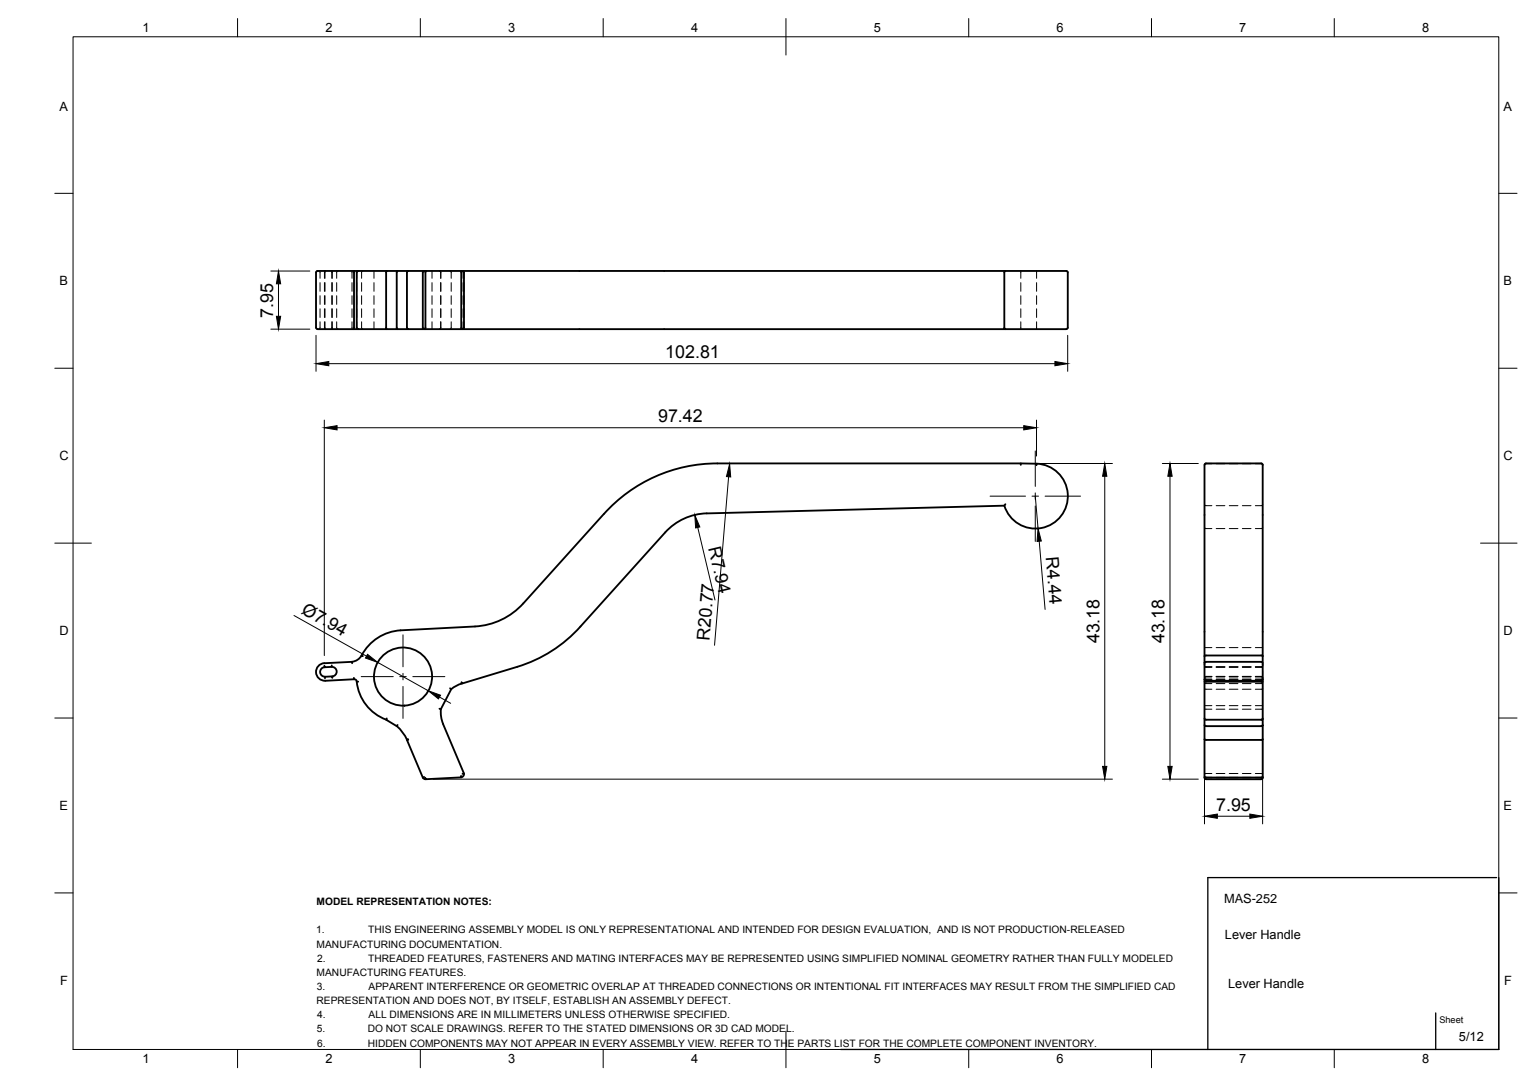
ISO-10303-21;
HEADER;
FILE_DESCRIPTION((''),'2;1');
FILE_NAME('Lever Handle.step','2026-10-06T07:01:46+05:00',(''),(''),'','','');
FILE_SCHEMA (('AUTOMOTIVE_DESIGN { 1 0 10303 214 3 1 1 }'));
ENDSEC;
DATA;
#10=MECHANICAL_DESIGN_GEOMETRIC_PRESENTATION_REPRESENTATION('',(#140),#11396);
#106=(
BOUNDED_SURFACE()
B_SPLINE_SURFACE(2,2,((#9482,#9483,#9484),(#9485,#9486,#9487),(#9488,#9489,
#9490)),.UNSPECIFIED.,.F.,.F.,.F.)
B_SPLINE_SURFACE_WITH_KNOTS((3,3),(3,3),(0.,1.5707963267949),(-2.95294089690097,
-1.43909013515432),.UNSPECIFIED.)
GEOMETRIC_REPRESENTATION_ITEM()
RATIONAL_B_SPLINE_SURFACE(((1.,0.726950752418356,1.),(0.707106781186548,
0.514031806623683,0.707106781186548),(1.,0.726950752418356,1.)))
REPRESENTATION_ITEM('')
SURFACE()
) ;
#107=(
BOUNDED_SURFACE()
B_SPLINE_SURFACE(2,2,((#10602,#10603,#10604),(#10605,#10606,#10607),(#10608,
#10609,#10610)),.UNSPECIFIED.,.F.,.F.,.F.)
B_SPLINE_SURFACE_WITH_KNOTS((3,3),(3,3),(-1.5707963267949,0.),(-2.95294089690006,
-1.43909013515442),.UNSPECIFIED.)
GEOMETRIC_REPRESENTATION_ITEM()
RATIONAL_B_SPLINE_SURFACE(((1.,0.726950752418703,1.),(0.707106781186561,
0.514031806623938,0.707106781186561),(1.,0.726950752418703,1.)))
REPRESENTATION_ITEM('')
SURFACE()
) ;
#110=SHAPE_REPRESENTATION_RELATIONSHIP('SRR','None',#11457,#125) ;
#125=ADVANCED_BREP_SHAPE_REPRESENTATION('',(#155),#11383) ;
#140=STYLED_ITEM('',(#11541),#155) ;
#155=MANIFOLD_SOLID_BREP('Lever Handle',#5571) ;
#202=TOROIDAL_SURFACE('',#6043,5.6095419988581,0.2) ;
#203=TOROIDAL_SURFACE('',#6047,18.7717409779691,0.2) ;
#204=TOROIDAL_SURFACE('',#6051,6.02789861439302,0.2) ;
#205=TOROIDAL_SURFACE('',#6055,0.524935224963979,0.2) ;
#206=TOROIDAL_SURFACE('',#6061,1.8962519345458,0.2) ;
#207=TOROIDAL_SURFACE('',#6064,20.567808830506,0.2) ;
#208=TOROIDAL_SURFACE('',#6067,6.24675996480776,0.2) ;
#209=TOROIDAL_SURFACE('',#6070,9.77267576253889,0.2) ;
#210=TOROIDAL_SURFACE('',#6077,1.00004201680672,0.2) ;
#211=TOROIDAL_SURFACE('',#6080,4.23606098801213,0.2) ;
#212=TOROIDAL_SURFACE('',#6084,8.13937148944777,0.2) ;
#213=TOROIDAL_SURFACE('',#6089,3.96067266925812,0.2) ;
#214=TOROIDAL_SURFACE('',#6093,4.37909654020415,0.2) ;
#215=TOROIDAL_SURFACE('',#6097,0.274381812079108,0.2) ;
#216=TOROIDAL_SURFACE('',#6128,0.274381812079108,0.2) ;
#217=TOROIDAL_SURFACE('',#6131,4.37909654020415,0.2) ;
#218=TOROIDAL_SURFACE('',#6135,3.96067266925812,0.2) ;
#219=TOROIDAL_SURFACE('',#6139,8.13937148944777,0.2) ;
#220=TOROIDAL_SURFACE('',#6144,1.00004201680672,0.2) ;
#221=TOROIDAL_SURFACE('',#6146,4.23606098801213,0.2) ;
#222=TOROIDAL_SURFACE('',#6151,9.77267576253889,0.2) ;
#223=TOROIDAL_SURFACE('',#6156,20.567808830506,0.2) ;
#224=TOROIDAL_SURFACE('',#6159,6.24675996480776,0.2) ;
#225=TOROIDAL_SURFACE('',#6162,1.8962519345458,0.2) ;
#226=TOROIDAL_SURFACE('',#6166,0.524935224963979,0.2) ;
#227=TOROIDAL_SURFACE('',#6169,18.7717409779691,0.2) ;
#228=TOROIDAL_SURFACE('',#6172,6.02789861439302,0.2) ;
#229=TOROIDAL_SURFACE('',#6175,5.6095419988581,0.2) ;
#230=TOROIDAL_SURFACE('',#6199,0.85017716535433,0.2) ;
#231=TOROIDAL_SURFACE('',#6202,0.85017716535433,0.2) ;
#232=TOROIDAL_SURFACE('',#6207,0.85017716535433,0.2) ;
#233=TOROIDAL_SURFACE('',#6209,0.85017716535433,0.2) ;
#271=B_SPLINE_CURVE_WITH_KNOTS('',3,(#9456,#9457,#9458,#9459,#9460,#9461,
#9462,#9463,#9464,#9465,#9466,#9467),.UNSPECIFIED.,.F.,.F.,(4,2,2,2,2,4),
(-0.000425934342717597,0.,0.00767782768113804,0.0154936481323793,0.0233033297268441,
0.0311102612476663),.UNSPECIFIED.) ;
#272=B_SPLINE_CURVE_WITH_KNOTS('',3,(#9470,#9471,#9472,#9473,#9474,#9475,
#9476,#9477,#9478,#9479,#9480,#9481),.UNSPECIFIED.,.F.,.F.,(4,2,2,2,2,4),
(-0.000392646763472729,0.,0.00776851635729194,0.0155945832419373,0.0233973193253328,
0.0311896776950334),.UNSPECIFIED.) ;
#273=B_SPLINE_CURVE_WITH_KNOTS('',3,(#9494,#9495,#9496,#9497,#9498,#9499,
#9500,#9501,#9502,#9503,#9504,#9505),.UNSPECIFIED.,.F.,.F.,(4,2,2,2,2,4),
(-0.0626678583597519,-0.0622419978775531,-0.0545506208202995,-0.046733489174686,
-0.0389252522766465,-0.0311209989394379),.UNSPECIFIED.) ;
#274=B_SPLINE_CURVE_WITH_KNOTS('',3,(#9511,#9512,#9513,#9514,#9515,#9516,
#9517,#9518,#9519,#9520,#9521,#9522),.UNSPECIFIED.,.F.,.F.,(4,2,2,2,2,4),
(-0.00029630356009181,0.,0.00778002873103429,0.0155932483092341,0.0234059593652307,
0.0312184094334333),.UNSPECIFIED.) ;
#275=B_SPLINE_CURVE_WITH_KNOTS('',3,(#9528,#9529,#9530,#9531,#9532,#9533,
#9534,#9535,#9536,#9537,#9538,#9539),.UNSPECIFIED.,.F.,.F.,(4,2,2,2,2,4),
(-0.0629385074257631,-0.0627334798904802,-0.0547568943966375,-0.046925593190769,
-0.0391229130222982,-0.0313664342990436),.UNSPECIFIED.) ;
#276=B_SPLINE_CURVE_WITH_KNOTS('',3,(#9545,#9546,#9547,#9548,#9549,#9550,
#9551,#9552,#9553,#9554,#9555,#9556),.UNSPECIFIED.,.F.,.F.,(4,2,2,2,2,4),
(-0.000203756697037429,0.,0.00796770405795475,0.0158037932485574,0.0236037819491495,
0.031385705039184),.UNSPECIFIED.) ;
#277=B_SPLINE_CURVE_WITH_KNOTS('',3,(#9561,#9562,#9563,#9564,#9565,#9566,
#9567,#9568,#9569,#9570,#9571,#9572,#9573,#9574,#9575,#9576,#9577,#9578,
#9579,#9580,#9581,#9582,#9583,#9584,#9585),.UNSPECIFIED.,.F.,.F.,(4,3,3,
3,3,3,3,3,4),(0.,0.199052542232163,0.398059502796862,0.597027074925485,
0.795961438809451,0.995008849549264,1.19397259651743,1.39300992499601,1.57079632692443),
 .UNSPECIFIED.) ;
#278=B_SPLINE_CURVE_WITH_KNOTS('',3,(#9589,#9590,#9591,#9592,#9593,#9594,
#9595,#9596,#9597,#9598,#9599,#9600),.UNSPECIFIED.,.F.,.F.,(4,2,2,2,2,4),
(-0.000302162807502731,0.,0.00777281639954654,0.0155857029470102,0.0233985882068449,
0.0312114728139599),.UNSPECIFIED.) ;
#279=B_SPLINE_CURVE_WITH_KNOTS('',3,(#9607,#9608,#9609,#9610,#9611,#9612,
#9613,#9614,#9615,#9616,#9617,#9618),.UNSPECIFIED.,.F.,.F.,(4,2,2,2,2,4),
(-0.0315148928540183,-0.0312005996265522,-0.0234381588919511,-0.0156248125751573,
-0.00781221363393156,0.),.UNSPECIFIED.) ;
#280=B_SPLINE_CURVE_WITH_KNOTS('',3,(#9623,#9624,#9625,#9626,#9627,#9628,
#9629,#9630,#9631,#9632,#9633,#9634),.UNSPECIFIED.,.F.,.F.,(4,2,2,2,2,4),
(-0.000209158996821947,0.,0.00790322324693375,0.0157271724669949,0.0235347393467978,
0.0313323503074072),.UNSPECIFIED.) ;
#281=B_SPLINE_CURVE_WITH_KNOTS('',3,(#9640,#9641,#9642,#9643,#9644,#9645,
#9646,#9647,#9648,#9649,#9650,#9651,#9652,#9653,#9654,#9655,#9656,#9657,
#9658,#9659,#9660,#9661,#9662,#9663,#9664),.UNSPECIFIED.,.F.,.F.,(4,3,3,
3,3,3,3,3,4),(0.,0.199052706978784,0.398059832253966,0.597027569062776,
0.7959620976022,0.99500967309516,1.19397358474941,1.39301107797699,1.57079762660799),
 .UNSPECIFIED.) ;
#282=B_SPLINE_CURVE_WITH_KNOTS('',3,(#9670,#9671,#9672,#9673,#9674,#9675,
#9676,#9677,#9678,#9679,#9680,#9681),.UNSPECIFIED.,.F.,.F.,(4,2,2,2,2,4),
(-0.000508786942166875,0.,0.00757813380105505,0.0153951238953111,0.0232058288277231,
0.0310129102887088),.UNSPECIFIED.) ;
#283=B_SPLINE_CURVE_WITH_KNOTS('',3,(#9686,#9687,#9688,#9689,#9690,#9691,
#9692,#9693,#9694,#9695,#9696,#9697,#9698,#9699,#9700,#9701,#9702,#9703,
#9704,#9705,#9706,#9707,#9708,#9709,#9710),.UNSPECIFIED.,.F.,.F.,(4,3,3,
3,3,3,3,3,4),(0.,0.199053248397837,0.398060914968089,0.597029192964828,
0.79596426260186,0.995012379499913,1.1939768323317,1.39301486693695,1.57080189914441),
 .UNSPECIFIED.) ;
#284=B_SPLINE_CURVE_WITH_KNOTS('',3,(#9714,#9715,#9716,#9717,#9718,#9719,
#9720,#9721,#9722,#9723,#9724,#9725,#9726,#9727,#9728,#9729),
 .UNSPECIFIED.,.F.,.F.,(4,2,2,2,2,2,2,4),(-0.00032358937009677,0.,0.00354444219611517,
0.00767686671153501,0.0154916858096829,0.0233035611079842,0.0311138771958668,
0.0311774645866534),.UNSPECIFIED.) ;
#285=B_SPLINE_CURVE_WITH_KNOTS('',3,(#9736,#9737,#9738,#9739,#9740,#9741,
#9742,#9743,#9744,#9745,#9746,#9747,#9748,#9749,#9750,#9751,#9752,#9753,
#9754,#9755,#9756,#9757,#9758,#9759,#9760),.UNSPECIFIED.,.F.,.F.,(4,3,3,
3,3,3,3,3,4),(0.,0.199052583563084,0.398059585450825,0.597027198896615,
0.795961604093608,0.99500905617405,1.19397284446766,1.39301021428897,1.57079665269337),
 .UNSPECIFIED.) ;
#286=B_SPLINE_CURVE_WITH_KNOTS('',3,(#9768,#9769,#9770,#9771,#9772,#9773,
#9774,#9775,#9776,#9777,#9778,#9779),.UNSPECIFIED.,.F.,.F.,(4,2,2,2,2,4),
(-0.0315123462948468,-0.031000483210486,-0.0234384406752481,-0.0156253470993035,
-0.00781258687358792,0.),.UNSPECIFIED.) ;
#287=B_SPLINE_CURVE_WITH_KNOTS('',3,(#9785,#9786,#9787,#9788,#9789,#9790,
#9791,#9792,#9793,#9794,#9795,#9796,#9797,#9798,#9799,#9800,#9801,#9802,
#9803,#9804,#9805,#9806,#9807,#9808,#9809),.UNSPECIFIED.,.F.,.F.,(4,3,3,
3,3,3,3,3,4),(0.,0.199052542245368,0.398059502823902,0.59702707496727,0.795961438867092,
0.9950088496244,1.19397259661093,1.39300992510867,1.57079632687287),
 .UNSPECIFIED.) ;
#288=B_SPLINE_CURVE_WITH_KNOTS('',3,(#9815,#9816,#9817,#9818,#9819,#9820,
#9821,#9822,#9823,#9824,#9825,#9826),.UNSPECIFIED.,.F.,.F.,(4,2,2,2,2,4),
(-0.000472807702419667,0.,0.00760072048225168,0.0154136353110866,0.0232265107396055,
0.0310393663455244),.UNSPECIFIED.) ;
#289=B_SPLINE_CURVE_WITH_KNOTS('',3,(#9831,#9832,#9833,#9834,#9835,#9836,
#9837,#9838,#9839,#9840,#9841,#9842,#9843,#9844,#9845,#9846,#9847,#9848,
#9849,#9850,#9851,#9852,#9853,#9854,#9855),.UNSPECIFIED.,.F.,.F.,(4,3,3,
3,3,3,3,3,4),(0.,0.199052542243981,0.398059502821061,0.597027074962877,
0.795961438861017,0.995008849616485,1.19397259660109,1.39300992509683,1.57079632687829),
 .UNSPECIFIED.) ;
#290=B_SPLINE_CURVE_WITH_KNOTS('',3,(#9872,#9873,#9874,#9875,#9876,#9877,
#9878,#9879,#9880,#9881,#9882,#9883),.UNSPECIFIED.,.F.,.F.,(4,2,2,2,2,4),
(-0.0315141126684919,-0.031176944954667,-0.0234383818709659,-0.0156252430234338,
-0.00781251789292829,0.),.UNSPECIFIED.) ;
#291=B_SPLINE_CURVE_WITH_KNOTS('',3,(#9887,#9888,#9889,#9890,#9891,#9892,
#9893,#9894,#9895,#9896,#9897,#9898,#9899,#9900,#9901,#9902,#9903,#9904,
#9905,#9906,#9907,#9908,#9909,#9910,#9911),.UNSPECIFIED.,.F.,.F.,(4,3,3,
3,3,3,3,3,4),(0.,0.199052485193076,0.398059386004224,0.597026894426605,
0.795961189880508,0.995008525064052,1.19397219273933,1.39300943847609,1.57079654966886),
 .UNSPECIFIED.) ;
#292=B_SPLINE_CURVE_WITH_KNOTS('',3,(#9919,#9920,#9921,#9922,#9923,#9924,
#9925,#9926,#9927,#9928,#9929,#9930,#9931,#9932),.UNSPECIFIED.,.F.,.F.,
(4,2,2,2,2,2,4),(-0.071485180683264,-0.0712307719726932,-0.064253173333706,
-0.0574900962687512,-0.0489313629526751,-0.0419539746827257,-0.0356153859867279),
 .UNSPECIFIED.) ;
#293=B_SPLINE_CURVE_WITH_KNOTS('',3,(#9950,#9951,#9952,#9953,#9954,#9955,
#9956,#9957,#9958,#9959,#9960,#9961,#9962,#9963),.UNSPECIFIED.,.F.,.F.,
(4,2,2,2,2,2,4),(-0.063419024433945,-0.0632138433555934,-0.0550363404792558,
-0.0471273977752151,-0.0393668335371398,-0.0316820163148599,-0.0316075730538707),
 .UNSPECIFIED.) ;
#294=B_SPLINE_CURVE_WITH_KNOTS('',3,(#9969,#9970,#9971,#9972,#9973,#9974,
#9975,#9976,#9977,#9978,#9979,#9980,#9981,#9982),.UNSPECIFIED.,.F.,.F.,
(4,2,2,2,2,2,4),(-0.000204835146312565,0.,0.00817143806143788,0.0160775285373022,
0.0238394400759123,0.0315278536559536,0.0315985683409222),.UNSPECIFIED.) ;
#295=B_SPLINE_CURVE_WITH_KNOTS('',3,(#9987,#9988,#9989,#9990,#9991,#9992,
#9993,#9994,#9995,#9996,#9997,#9998,#9999,#10000),.UNSPECIFIED.,.F.,.F.,
(4,2,2,2,2,2,4),(-0.0315119651507534,-0.0310369720406695,-0.0234522322979694,
-0.0156393394528541,-0.00782644846731675,-1.35584415946594E-5,0.),
 .UNSPECIFIED.) ;
#296=B_SPLINE_CURVE_WITH_KNOTS('',3,(#10007,#10008,#10009,#10010,#10011,
#10012,#10013,#10014,#10015,#10016,#10017,#10018),.UNSPECIFIED.,.F.,.F.,
(4,2,2,2,2,4),(-0.031721691652862,-0.0314189347322439,-0.0233633267396854,
-0.0155133765946492,-0.00773979585571865,0.),.UNSPECIFIED.) ;
#297=B_SPLINE_CURVE_WITH_KNOTS('',3,(#10099,#10100,#10101,#10102,#10103,
#10104,#10105,#10106,#10107,#10108,#10109,#10110),.UNSPECIFIED.,.F.,.F.,
(4,2,2,2,2,4),(-0.000302979244329871,0.,0.00806152347440571,0.0159172380801614,
0.0236965271994009,0.0314420066261495),.UNSPECIFIED.) ;
#298=B_SPLINE_CURVE_WITH_KNOTS('',3,(#10111,#10112,#10113,#10114,#10115,
#10116,#10117,#10118,#10119,#10120,#10121,#10122),.UNSPECIFIED.,.F.,.F.,
(4,2,2,2,2,4),(-0.0315754136058091,-0.0311828527614278,-0.0234160363129251,
-0.0155916819303375,-0.00779065324374899,0.),.UNSPECIFIED.) ;
#299=B_SPLINE_CURVE_WITH_KNOTS('',3,(#10127,#10128,#10129,#10130,#10131,
#10132,#10133,#10134,#10135,#10136,#10137,#10138,#10139,#10140),
 .UNSPECIFIED.,.F.,.F.,(4,2,2,2,2,2,4),(-0.000474992982336123,0.,0.00758473725973339,
0.0153976269864644,0.0232105148526209,0.0310234017590763,0.0310369601957522),
 .UNSPECIFIED.) ;
#300=B_SPLINE_CURVE_WITH_KNOTS('',3,(#10146,#10147,#10148,#10149,#10150,
#10151,#10152,#10153,#10154,#10155,#10156,#10157),.UNSPECIFIED.,.F.,.F.,
(4,2,2,2,2,4),(-0.0634032075025796,-0.0631983745559419,-0.0551219653781809,
-0.0471164301307063,-0.039256298781182,-0.0315985683616453),
 .UNSPECIFIED.) ;
#301=B_SPLINE_CURVE_WITH_KNOTS('',3,(#10163,#10164,#10165,#10166,#10167,
#10168,#10169,#10170,#10171,#10172,#10173,#10174),.UNSPECIFIED.,.F.,.F.,
(4,2,2,2,2,4),(-0.000205178731636372,0.,0.00808313825878162,0.0160941684934645,
0.0239559117961846,0.0316075730471855),.UNSPECIFIED.) ;
#302=B_SPLINE_CURVE_WITH_KNOTS('',3,(#10180,#10181,#10182,#10183,#10184,
#10185,#10186,#10187,#10188,#10189,#10190,#10191),.UNSPECIFIED.,.F.,.F.,
(4,2,2,2,2,4),(-0.000314294385248188,0.,0.00776246933425461,0.0155758444397962,
0.0233884721670194,0.0312007145855276),.UNSPECIFIED.) ;
#303=B_SPLINE_CURVE_WITH_KNOTS('',3,(#10195,#10196,#10197,#10198,#10199,
#10200,#10201,#10202,#10203,#10204,#10205,#10206,#10207,#10208,#10209,#10210,
#10211,#10212,#10213,#10214,#10215,#10216,#10217,#10218,#10219),
 .UNSPECIFIED.,.F.,.F.,(4,3,3,3,3,3,3,3,4),(0.,0.199053248397837,0.398060914968088,
0.597029192964836,0.795964262601867,0.995012379499923,1.19397683233171,
1.39301486693695,1.57080189914441),.UNSPECIFIED.) ;
#304=B_SPLINE_CURVE_WITH_KNOTS('',3,(#10222,#10223,#10224,#10225,#10226,
#10227,#10228,#10229,#10230,#10231,#10232,#10233),.UNSPECIFIED.,.F.,.F.,
(4,2,2,2,2,4),(-0.0315210097541554,-0.0310122339084761,-0.0234342653837737,
-0.0156174457752067,-0.00780691119140275,0.),.UNSPECIFIED.) ;
#305=B_SPLINE_CURVE_WITH_KNOTS('',3,(#10237,#10238,#10239,#10240,#10241,
#10242,#10243,#10244,#10245,#10246,#10247,#10248,#10249,#10250,#10251,#10252,
#10253,#10254,#10255,#10256,#10257,#10258,#10259,#10260,#10261),
 .UNSPECIFIED.,.F.,.F.,(4,3,3,3,3,3,3,3,4),(0.,0.199052542064369,0.398059502453293,
0.597027074394497,0.795961438077169,0.995008848594717,1.19397259532962,
1.39300992356481,1.57079632757971),.UNSPECIFIED.) ;
#306=B_SPLINE_CURVE_WITH_KNOTS('',3,(#10272,#10273,#10274,#10275,#10276,
#10277,#10278,#10279,#10280,#10281,#10282,#10283,#10284,#10285),
 .UNSPECIFIED.,.F.,.F.,(4,2,2,2,2,2,4),(-0.000254408710349561,0.,0.00697759863796767,
0.0137406757011616,0.0222994090150433,0.0292767972832062,0.035615385977577),
 .UNSPECIFIED.) ;
#307=B_SPLINE_CURVE_WITH_KNOTS('',3,(#10288,#10289,#10290,#10291,#10292,
#10293,#10294,#10295,#10296,#10297,#10298,#10299,#10300,#10301,#10302,#10303,
#10304,#10305,#10306,#10307,#10308,#10309,#10310,#10311,#10312),
 .UNSPECIFIED.,.F.,.F.,(4,3,3,3,3,3,3,3,4),(0.,0.199052485193076,0.398059386004222,
0.597026894426605,0.795961189880508,0.995008525064048,1.19397219273933,
1.39300943847609,1.57079654966886),.UNSPECIFIED.) ;
#308=B_SPLINE_CURVE_WITH_KNOTS('',3,(#10318,#10319,#10320,#10321,#10322,
#10323,#10324,#10325,#10326,#10327,#10328,#10329),.UNSPECIFIED.,.F.,.F.,
(4,2,2,2,2,4),(-0.000337168458022535,0.,0.00773858016387553,0.0155517362556591,
0.0233644786295,0.031177013765312),.UNSPECIFIED.) ;
#309=B_SPLINE_CURVE_WITH_KNOTS('',3,(#10339,#10340,#10341,#10342,#10343,
#10344,#10345,#10346,#10347,#10348,#10349,#10350,#10351,#10352,#10353,#10354,
#10355,#10356,#10357,#10358,#10359,#10360,#10361,#10362,#10363),
 .UNSPECIFIED.,.F.,.F.,(4,3,3,3,3,3,3,3,4),(0.,0.199052542234199,0.398059502803477,
0.597027074940396,0.795961438837137,0.995008849596832,1.1939725965883,1.39300992509389,
1.57079632687829),.UNSPECIFIED.) ;
#310=B_SPLINE_CURVE_WITH_KNOTS('',3,(#10370,#10371,#10372,#10373,#10374,
#10375,#10376,#10377,#10378,#10379,#10380,#10381,#10382,#10383,#10384,#10385,
#10386,#10387,#10388,#10389,#10390,#10391,#10392,#10393,#10394),
 .UNSPECIFIED.,.F.,.F.,(4,3,3,3,3,3,3,3,4),(0.,0.199052646770473,0.398059711851129,
0.597027388477328,0.795961856844187,0.99500937213039,1.19397322360319,1.39301065662705,
1.5707971514832),.UNSPECIFIED.) ;
#311=B_SPLINE_CURVE_WITH_KNOTS('',3,(#10400,#10401,#10402,#10403,#10404,
#10405,#10406,#10407,#10408,#10409,#10410,#10411),.UNSPECIFIED.,.F.,.F.,
(4,2,2,2,2,4),(-0.0315121677712463,-0.0310393601655826,-0.0234386412048373,
-0.0156257279288386,-0.00781285405311264,0.),.UNSPECIFIED.) ;
#312=B_SPLINE_CURVE_WITH_KNOTS('',3,(#10415,#10416,#10417,#10418,#10419,
#10420,#10421,#10422,#10423,#10424,#10425,#10426,#10427,#10428,#10429,#10430,
#10431,#10432,#10433,#10434,#10435,#10436,#10437,#10438,#10439),
 .UNSPECIFIED.,.F.,.F.,(4,3,3,3,3,3,3,3,4),(0.,0.199052542257445,0.39805950284863,
0.597027075005487,0.795961438919784,0.995008849693087,1.1939725966964,1.39300992521166,
1.57079632682576),.UNSPECIFIED.) ;
#313=B_SPLINE_CURVE_WITH_KNOTS('',3,(#10445,#10446,#10447,#10448,#10449,
#10450,#10451,#10452,#10453,#10454,#10455,#10456),.UNSPECIFIED.,.F.,.F.,
(4,2,2,2,2,4),(-0.0315141739942469,-0.031204434348752,-0.0234384419466034,
-0.0156253478250137,-0.00781258702147206,0.),.UNSPECIFIED.) ;
#314=B_SPLINE_CURVE_WITH_KNOTS('',3,(#10463,#10464,#10465,#10466,#10467,
#10468,#10469,#10470,#10471,#10472,#10473,#10474),.UNSPECIFIED.,.F.,.F.,
(4,2,2,2,2,4),(-0.0626970871191847,-0.0623734982158925,-0.054555633082751,
-0.0467389670549674,-0.0389250691737583,-0.0311774645911791),
 .UNSPECIFIED.) ;
#315=B_SPLINE_CURVE_WITH_KNOTS('',3,(#10480,#10481,#10482,#10483,#10484,
#10485,#10486,#10487,#10488,#10489,#10490,#10491,#10492,#10493,#10494,#10495,
#10496,#10497,#10498,#10499,#10500,#10501,#10502,#10503,#10504),
 .UNSPECIFIED.,.F.,.F.,(4,3,3,3,3,3,3,3,4),(0.,0.199052686881998,0.398059792064997,
0.597027508785601,0.795962017240172,0.995009572636864,1.1939734642033,1.39301093733562,
1.57079746801826),.UNSPECIFIED.) ;
#316=B_SPLINE_CURVE_WITH_KNOTS('',3,(#10510,#10511,#10512,#10513,#10514,
#10515,#10516,#10517,#10518,#10519,#10520,#10521),.UNSPECIFIED.,.F.,.F.,
(4,2,2,2,2,4),(-0.000404724526048245,0.,0.00770679420177707,0.015530569118343,
0.0233375581471532,0.0311349644051186),.UNSPECIFIED.) ;
#317=B_SPLINE_CURVE_WITH_KNOTS('',3,(#10526,#10527,#10528,#10529,#10530,
#10531,#10532,#10533,#10534,#10535,#10536,#10537),.UNSPECIFIED.,.F.,.F.,
(4,2,2,2,2,4),(-0.0315136505422076,-0.0312114875916089,-0.0234386675146469,
-0.0156257772666477,-0.00781288830710044,0.),.UNSPECIFIED.) ;
#318=B_SPLINE_CURVE_WITH_KNOTS('',3,(#10545,#10546,#10547,#10548,#10549,
#10550,#10551,#10552,#10553,#10554,#10555,#10556),.UNSPECIFIED.,.F.,.F.,
(4,2,2,2,2,4),(-0.0629751667751677,-0.0627714100781202,-0.0548037060202023,
-0.0469676168296412,-0.0391676281290893,-0.0313857050390938),
 .UNSPECIFIED.) ;
#319=B_SPLINE_CURVE_WITH_KNOTS('',3,(#10560,#10561,#10562,#10563,#10564,
#10565,#10566,#10567,#10568,#10569,#10570,#10571),.UNSPECIFIED.,.F.,.F.,
(4,2,2,2,2,4),(-0.00020502755219765,0.,0.00797658615153273,0.015807888001696,
0.0236105688121075,0.031367048172),.UNSPECIFIED.) ;
#320=B_SPLINE_CURVE_WITH_KNOTS('',3,(#10575,#10576,#10577,#10578,#10579,
#10580,#10581,#10582,#10583,#10584,#10585,#10586),.UNSPECIFIED.,.F.,.F.,
(4,2,2,2,2,4),(-0.0315146329369706,-0.0312183301295434,-0.0234383211620277,
-0.0156251214317014,-0.00781243022228811,0.),.UNSPECIFIED.) ;
#321=B_SPLINE_CURVE_WITH_KNOTS('',3,(#10590,#10591,#10592,#10593,#10594,
#10595,#10596,#10597,#10598,#10599,#10600,#10601),.UNSPECIFIED.,.F.,.F.,
(4,2,2,2,2,4),(-0.00042586048217451,0.,0.00769137706195492,0.0155085087115375,
0.0233167456135432,0.0311209989547217),.UNSPECIFIED.) ;
#322=B_SPLINE_CURVE_WITH_KNOTS('',3,(#10613,#10614,#10615,#10616,#10617,
#10618,#10619,#10620,#10621,#10622,#10623,#10624),.UNSPECIFIED.,.F.,.F.,
(4,2,2,2,2,4),(-0.0626464568378844,-0.0622205224951688,-0.0545426948140428,
-0.0467268743628218,-0.038917192768381,-0.0311102612475827),
 .UNSPECIFIED.) ;
#323=B_SPLINE_CURVE_WITH_KNOTS('',3,(#10667,#10668,#10669,#10670,#10671,
#10672,#10673,#10674,#10675,#10676,#10677,#10678),.UNSPECIFIED.,.F.,.F.,
(4,2,2,2,2,4),(-0.000583318373026515,0.,0.00749040753634202,0.0153036497211779,
0.0231163526509165,0.0309287602356685),.UNSPECIFIED.) ;
#324=B_SPLINE_CURVE_WITH_KNOTS('',3,(#10681,#10682,#10683,#10684,#10685,
#10686,#10687,#10688,#10689,#10690,#10691,#10692),.UNSPECIFIED.,.F.,.F.,
(4,2,2,2,2,4),(-0.0315120082952079,-0.0309286912237509,-0.0234383004008955,
-0.0156250756498918,-0.00781239015278319,0.),.UNSPECIFIED.) ;
#325=B_SPLINE_CURVE_WITH_KNOTS('',3,(#10695,#10696,#10697,#10698,#10699,
#10700,#10701,#10702,#10703,#10704,#10705,#10706),.UNSPECIFIED.,.F.,.F.,
(4,2,2,2,2,4),(-0.0315120082952136,-0.0309286912237554,-0.0234383004008859,
-0.0156250756498869,-0.0078123901527818,0.),.UNSPECIFIED.) ;
#326=B_SPLINE_CURVE_WITH_KNOTS('',3,(#10710,#10711,#10712,#10713,#10714,
#10715,#10716,#10717,#10718,#10719,#10720,#10721),.UNSPECIFIED.,.F.,.F.,
(4,2,2,2,2,4),(-0.000583318373025772,0.,0.0074904075363243,0.0153036497211384,
0.0231163526508542,0.0309287602355855),.UNSPECIFIED.) ;
#327=B_SPLINE_CURVE_WITH_KNOTS('',3,(#10738,#10739,#10740,#10741,#10742,
#10743,#10744,#10745,#10746,#10747,#10748,#10749),.UNSPECIFIED.,.F.,.F.,
(4,2,2,2,2,4),(-0.030928760235604,-0.0231163526508699,-0.0153036497211549,
-0.00749040753633595,0.,0.000583318373037331),.UNSPECIFIED.) ;
#328=B_SPLINE_CURVE_WITH_KNOTS('',3,(#10750,#10751,#10752,#10753,#10754,
#10755,#10756,#10757,#10758,#10759,#10760,#10761),.UNSPECIFIED.,.F.,.F.,
(4,2,2,2,2,4),(-0.0315120082952245,-0.0309286912237537,-0.0234383004008807,
-0.0156250756498813,-0.00781239015277872,0.),.UNSPECIFIED.) ;
#329=B_SPLINE_CURVE_WITH_KNOTS('',3,(#10763,#10764,#10765,#10766,#10767,
#10768,#10769,#10770,#10771,#10772,#10773,#10774),.UNSPECIFIED.,.F.,.F.,
(4,2,2,2,2,4),(-0.0315120082952178,-0.0309286912237491,-0.0234383004008884,
-0.0156250756498874,-0.00781239015278138,0.),.UNSPECIFIED.) ;
#330=B_SPLINE_CURVE_WITH_KNOTS('',3,(#10775,#10776,#10777,#10778,#10779,
#10780,#10781,#10782,#10783,#10784,#10785,#10786),.UNSPECIFIED.,.F.,.F.,
(4,2,2,2,2,4),(-0.00058331837303795,0.,0.00749040753635054,0.0153036497211894,
0.0231163526509301,0.0309287602356871),.UNSPECIFIED.) ;
#359=FACE_BOUND('',#1053,.T.) ;
#360=FACE_BOUND('',#1054,.T.) ;
#361=FACE_BOUND('',#1099,.T.) ;
#362=FACE_BOUND('',#1100,.T.) ;
#394=ELLIPSE('',#6060,0.200007949139568,0.2) ;
#395=ELLIPSE('',#6150,0.200007949139572,0.2) ;
#442=PLANE('',#6102) ;
#443=PLANE('',#6105) ;
#444=PLANE('',#6108) ;
#445=PLANE('',#6113) ;
#446=PLANE('',#6116) ;
#447=PLANE('',#6121) ;
#448=PLANE('',#6124) ;
#449=PLANE('',#6180) ;
#450=PLANE('',#6182) ;
#451=PLANE('',#6184) ;
#452=PLANE('',#6186) ;
#453=PLANE('',#6188) ;
#454=PLANE('',#6190) ;
#455=PLANE('',#6191) ;
#456=PLANE('',#6193) ;
#457=PLANE('',#6194) ;
#458=PLANE('',#6206) ;
#459=PLANE('',#6213) ;
#650=FACE_OUTER_BOUND('',#1008,.T.) ;
#651=FACE_OUTER_BOUND('',#1009,.T.) ;
#652=FACE_OUTER_BOUND('',#1010,.T.) ;
#653=FACE_OUTER_BOUND('',#1011,.T.) ;
#654=FACE_OUTER_BOUND('',#1012,.T.) ;
#655=FACE_OUTER_BOUND('',#1013,.T.) ;
#656=FACE_OUTER_BOUND('',#1014,.T.) ;
#657=FACE_OUTER_BOUND('',#1015,.T.) ;
#658=FACE_OUTER_BOUND('',#1016,.T.) ;
#659=FACE_OUTER_BOUND('',#1017,.T.) ;
#660=FACE_OUTER_BOUND('',#1018,.T.) ;
#661=FACE_OUTER_BOUND('',#1019,.T.) ;
#662=FACE_OUTER_BOUND('',#1020,.T.) ;
#663=FACE_OUTER_BOUND('',#1021,.T.) ;
#664=FACE_OUTER_BOUND('',#1022,.T.) ;
#665=FACE_OUTER_BOUND('',#1023,.T.) ;
#666=FACE_OUTER_BOUND('',#1024,.T.) ;
#667=FACE_OUTER_BOUND('',#1025,.T.) ;
#668=FACE_OUTER_BOUND('',#1026,.T.) ;
#669=FACE_OUTER_BOUND('',#1027,.T.) ;
#670=FACE_OUTER_BOUND('',#1028,.T.) ;
#671=FACE_OUTER_BOUND('',#1029,.T.) ;
#672=FACE_OUTER_BOUND('',#1030,.T.) ;
#673=FACE_OUTER_BOUND('',#1031,.T.) ;
#674=FACE_OUTER_BOUND('',#1032,.T.) ;
#675=FACE_OUTER_BOUND('',#1033,.T.) ;
#676=FACE_OUTER_BOUND('',#1034,.T.) ;
#677=FACE_OUTER_BOUND('',#1035,.T.) ;
#678=FACE_OUTER_BOUND('',#1036,.T.) ;
#679=FACE_OUTER_BOUND('',#1037,.T.) ;
#680=FACE_OUTER_BOUND('',#1038,.T.) ;
#681=FACE_OUTER_BOUND('',#1039,.T.) ;
#682=FACE_OUTER_BOUND('',#1040,.T.) ;
#683=FACE_OUTER_BOUND('',#1041,.T.) ;
#684=FACE_OUTER_BOUND('',#1042,.T.) ;
#685=FACE_OUTER_BOUND('',#1043,.T.) ;
#686=FACE_OUTER_BOUND('',#1044,.T.) ;
#687=FACE_OUTER_BOUND('',#1045,.T.) ;
#688=FACE_OUTER_BOUND('',#1046,.T.) ;
#689=FACE_OUTER_BOUND('',#1047,.T.) ;
#690=FACE_OUTER_BOUND('',#1048,.T.) ;
#691=FACE_OUTER_BOUND('',#1049,.T.) ;
#692=FACE_OUTER_BOUND('',#1050,.T.) ;
#693=FACE_OUTER_BOUND('',#1051,.T.) ;
#694=FACE_OUTER_BOUND('',#1052,.T.) ;
#695=FACE_OUTER_BOUND('',#1055,.T.) ;
#696=FACE_OUTER_BOUND('',#1056,.T.) ;
#697=FACE_OUTER_BOUND('',#1057,.T.) ;
#698=FACE_OUTER_BOUND('',#1058,.T.) ;
#699=FACE_OUTER_BOUND('',#1059,.T.) ;
#700=FACE_OUTER_BOUND('',#1060,.T.) ;
#701=FACE_OUTER_BOUND('',#1061,.T.) ;
#702=FACE_OUTER_BOUND('',#1062,.T.) ;
#703=FACE_OUTER_BOUND('',#1063,.T.) ;
#704=FACE_OUTER_BOUND('',#1064,.T.) ;
#705=FACE_OUTER_BOUND('',#1065,.T.) ;
#706=FACE_OUTER_BOUND('',#1066,.T.) ;
#707=FACE_OUTER_BOUND('',#1067,.T.) ;
#708=FACE_OUTER_BOUND('',#1068,.T.) ;
#709=FACE_OUTER_BOUND('',#1069,.T.) ;
#710=FACE_OUTER_BOUND('',#1070,.T.) ;
#711=FACE_OUTER_BOUND('',#1071,.T.) ;
#712=FACE_OUTER_BOUND('',#1072,.T.) ;
#713=FACE_OUTER_BOUND('',#1073,.T.) ;
#714=FACE_OUTER_BOUND('',#1074,.T.) ;
#715=FACE_OUTER_BOUND('',#1075,.T.) ;
#716=FACE_OUTER_BOUND('',#1076,.T.) ;
#717=FACE_OUTER_BOUND('',#1077,.T.) ;
#718=FACE_OUTER_BOUND('',#1078,.T.) ;
#719=FACE_OUTER_BOUND('',#1079,.T.) ;
#720=FACE_OUTER_BOUND('',#1080,.T.) ;
#721=FACE_OUTER_BOUND('',#1081,.T.) ;
#722=FACE_OUTER_BOUND('',#1082,.T.) ;
#723=FACE_OUTER_BOUND('',#1083,.T.) ;
#724=FACE_OUTER_BOUND('',#1084,.T.) ;
#725=FACE_OUTER_BOUND('',#1085,.T.) ;
#726=FACE_OUTER_BOUND('',#1086,.T.) ;
#727=FACE_OUTER_BOUND('',#1087,.T.) ;
#728=FACE_OUTER_BOUND('',#1088,.T.) ;
#729=FACE_OUTER_BOUND('',#1089,.T.) ;
#730=FACE_OUTER_BOUND('',#1090,.T.) ;
#731=FACE_OUTER_BOUND('',#1091,.T.) ;
#732=FACE_OUTER_BOUND('',#1092,.T.) ;
#733=FACE_OUTER_BOUND('',#1093,.T.) ;
#734=FACE_OUTER_BOUND('',#1094,.T.) ;
#735=FACE_OUTER_BOUND('',#1095,.T.) ;
#736=FACE_OUTER_BOUND('',#1096,.T.) ;
#737=FACE_OUTER_BOUND('',#1097,.T.) ;
#738=FACE_OUTER_BOUND('',#1098,.T.) ;
#739=FACE_OUTER_BOUND('',#1101,.T.) ;
#740=FACE_OUTER_BOUND('',#1102,.T.) ;
#741=FACE_OUTER_BOUND('',#1103,.T.) ;
#742=FACE_OUTER_BOUND('',#1104,.T.) ;
#743=FACE_OUTER_BOUND('',#1105,.T.) ;
#744=FACE_OUTER_BOUND('',#1106,.T.) ;
#745=FACE_OUTER_BOUND('',#1107,.T.) ;
#746=FACE_OUTER_BOUND('',#1108,.T.) ;
#747=FACE_OUTER_BOUND('',#1109,.T.) ;
#748=FACE_OUTER_BOUND('',#1110,.T.) ;
#749=FACE_OUTER_BOUND('',#1111,.T.) ;
#750=FACE_OUTER_BOUND('',#1112,.T.) ;
#751=FACE_OUTER_BOUND('',#1113,.T.) ;
#1008=EDGE_LOOP('',(#4244,#4245,#4246,#4247)) ;
#1009=EDGE_LOOP('',(#4248,#4249,#4250,#4251)) ;
#1010=EDGE_LOOP('',(#4252,#4253,#4254,#4255)) ;
#1011=EDGE_LOOP('',(#4256,#4257,#4258,#4259)) ;
#1012=EDGE_LOOP('',(#4260,#4261,#4262,#4263)) ;
#1013=EDGE_LOOP('',(#4264,#4265,#4266,#4267)) ;
#1014=EDGE_LOOP('',(#4268,#4269,#4270,#4271)) ;
#1015=EDGE_LOOP('',(#4272,#4273,#4274,#4275)) ;
#1016=EDGE_LOOP('',(#4276,#4277,#4278,#4279)) ;
#1017=EDGE_LOOP('',(#4280,#4281,#4282,#4283)) ;
#1018=EDGE_LOOP('',(#4284,#4285,#4286,#4287)) ;
#1019=EDGE_LOOP('',(#4288,#4289,#4290,#4291)) ;
#1020=EDGE_LOOP('',(#4292,#4293,#4294,#4295)) ;
#1021=EDGE_LOOP('',(#4296,#4297,#4298,#4299)) ;
#1022=EDGE_LOOP('',(#4300,#4301,#4302,#4303)) ;
#1023=EDGE_LOOP('',(#4304,#4305,#4306,#4307)) ;
#1024=EDGE_LOOP('',(#4308,#4309,#4310,#4311)) ;
#1025=EDGE_LOOP('',(#4312,#4313,#4314,#4315)) ;
#1026=EDGE_LOOP('',(#4316,#4317,#4318,#4319)) ;
#1027=EDGE_LOOP('',(#4320,#4321,#4322,#4323)) ;
#1028=EDGE_LOOP('',(#4324,#4325,#4326,#4327)) ;
#1029=EDGE_LOOP('',(#4328,#4329,#4330,#4331)) ;
#1030=EDGE_LOOP('',(#4332,#4333,#4334,#4335)) ;
#1031=EDGE_LOOP('',(#4336,#4337,#4338,#4339)) ;
#1032=EDGE_LOOP('',(#4340,#4341,#4342,#4343)) ;
#1033=EDGE_LOOP('',(#4344,#4345,#4346,#4347)) ;
#1034=EDGE_LOOP('',(#4348,#4349,#4350,#4351)) ;
#1035=EDGE_LOOP('',(#4352,#4353,#4354,#4355)) ;
#1036=EDGE_LOOP('',(#4356,#4357,#4358,#4359)) ;
#1037=EDGE_LOOP('',(#4360,#4361,#4362,#4363)) ;
#1038=EDGE_LOOP('',(#4364,#4365,#4366,#4367)) ;
#1039=EDGE_LOOP('',(#4368,#4369,#4370,#4371)) ;
#1040=EDGE_LOOP('',(#4372,#4373,#4374,#4375)) ;
#1041=EDGE_LOOP('',(#4376,#4377,#4378,#4379)) ;
#1042=EDGE_LOOP('',(#4380,#4381,#4382,#4383)) ;
#1043=EDGE_LOOP('',(#4384,#4385,#4386,#4387)) ;
#1044=EDGE_LOOP('',(#4388,#4389,#4390,#4391)) ;
#1045=EDGE_LOOP('',(#4392,#4393,#4394,#4395)) ;
#1046=EDGE_LOOP('',(#4396,#4397,#4398,#4399)) ;
#1047=EDGE_LOOP('',(#4400,#4401,#4402,#4403)) ;
#1048=EDGE_LOOP('',(#4404,#4405,#4406,#4407)) ;
#1049=EDGE_LOOP('',(#4408,#4409,#4410,#4411)) ;
#1050=EDGE_LOOP('',(#4412,#4413,#4414,#4415)) ;
#1051=EDGE_LOOP('',(#4416,#4417,#4418,#4419)) ;
#1052=EDGE_LOOP('',(#4420,#4421,#4422,#4423,#4424,#4425,#4426,#4427,#4428,
#4429,#4430,#4431,#4432,#4433,#4434,#4435,#4436,#4437,#4438,#4439,#4440,
#4441,#4442,#4443,#4444,#4445,#4446,#4447,#4448)) ;
#1053=EDGE_LOOP('',(#4449,#4450,#4451,#4452)) ;
#1054=EDGE_LOOP('',(#4453)) ;
#1055=EDGE_LOOP('',(#4454,#4455,#4456,#4457)) ;
#1056=EDGE_LOOP('',(#4458,#4459,#4460,#4461)) ;
#1057=EDGE_LOOP('',(#4462,#4463,#4464,#4465)) ;
#1058=EDGE_LOOP('',(#4466,#4467,#4468,#4469)) ;
#1059=EDGE_LOOP('',(#4470,#4471,#4472,#4473)) ;
#1060=EDGE_LOOP('',(#4474,#4475,#4476,#4477)) ;
#1061=EDGE_LOOP('',(#4478,#4479,#4480,#4481)) ;
#1062=EDGE_LOOP('',(#4482,#4483,#4484,#4485)) ;
#1063=EDGE_LOOP('',(#4486,#4487,#4488,#4489)) ;
#1064=EDGE_LOOP('',(#4490,#4491,#4492,#4493)) ;
#1065=EDGE_LOOP('',(#4494,#4495,#4496,#4497)) ;
#1066=EDGE_LOOP('',(#4498,#4499,#4500,#4501)) ;
#1067=EDGE_LOOP('',(#4502,#4503,#4504,#4505)) ;
#1068=EDGE_LOOP('',(#4506,#4507,#4508,#4509)) ;
#1069=EDGE_LOOP('',(#4510,#4511,#4512,#4513)) ;
#1070=EDGE_LOOP('',(#4514,#4515,#4516,#4517)) ;
#1071=EDGE_LOOP('',(#4518,#4519,#4520,#4521)) ;
#1072=EDGE_LOOP('',(#4522,#4523,#4524,#4525)) ;
#1073=EDGE_LOOP('',(#4526,#4527,#4528,#4529)) ;
#1074=EDGE_LOOP('',(#4530,#4531,#4532,#4533)) ;
#1075=EDGE_LOOP('',(#4534,#4535,#4536,#4537)) ;
#1076=EDGE_LOOP('',(#4538,#4539,#4540,#4541)) ;
#1077=EDGE_LOOP('',(#4542,#4543,#4544,#4545)) ;
#1078=EDGE_LOOP('',(#4546,#4547,#4548,#4549)) ;
#1079=EDGE_LOOP('',(#4550,#4551,#4552,#4553)) ;
#1080=EDGE_LOOP('',(#4554,#4555,#4556,#4557)) ;
#1081=EDGE_LOOP('',(#4558,#4559,#4560,#4561)) ;
#1082=EDGE_LOOP('',(#4562,#4563,#4564,#4565)) ;
#1083=EDGE_LOOP('',(#4566,#4567,#4568,#4569)) ;
#1084=EDGE_LOOP('',(#4570,#4571,#4572,#4573)) ;
#1085=EDGE_LOOP('',(#4574,#4575,#4576,#4577)) ;
#1086=EDGE_LOOP('',(#4578,#4579,#4580,#4581)) ;
#1087=EDGE_LOOP('',(#4582,#4583,#4584,#4585)) ;
#1088=EDGE_LOOP('',(#4586,#4587,#4588,#4589)) ;
#1089=EDGE_LOOP('',(#4590,#4591,#4592,#4593)) ;
#1090=EDGE_LOOP('',(#4594,#4595,#4596,#4597)) ;
#1091=EDGE_LOOP('',(#4598,#4599,#4600,#4601)) ;
#1092=EDGE_LOOP('',(#4602,#4603,#4604,#4605)) ;
#1093=EDGE_LOOP('',(#4606,#4607,#4608,#4609)) ;
#1094=EDGE_LOOP('',(#4610,#4611,#4612,#4613)) ;
#1095=EDGE_LOOP('',(#4614,#4615,#4616,#4617)) ;
#1096=EDGE_LOOP('',(#4618,#4619,#4620,#4621)) ;
#1097=EDGE_LOOP('',(#4622,#4623,#4624,#4625)) ;
#1098=EDGE_LOOP('',(#4626,#4627,#4628,#4629,#4630,#4631,#4632,#4633,#4634,
#4635,#4636,#4637,#4638,#4639,#4640,#4641,#4642,#4643,#4644,#4645,#4646,
#4647,#4648,#4649,#4650,#4651,#4652,#4653,#4654)) ;
#1099=EDGE_LOOP('',(#4655,#4656,#4657,#4658)) ;
#1100=EDGE_LOOP('',(#4659)) ;
#1101=EDGE_LOOP('',(#4660,#4661,#4662,#4663)) ;
#1102=EDGE_LOOP('',(#4664,#4665,#4666,#4667)) ;
#1103=EDGE_LOOP('',(#4668,#4669,#4670,#4671)) ;
#1104=EDGE_LOOP('',(#4672,#4673,#4674,#4675)) ;
#1105=EDGE_LOOP('',(#4676,#4677,#4678,#4679)) ;
#1106=EDGE_LOOP('',(#4680,#4681,#4682,#4683)) ;
#1107=EDGE_LOOP('',(#4684,#4685,#4686,#4687)) ;
#1108=EDGE_LOOP('',(#4688,#4689,#4690,#4691)) ;
#1109=EDGE_LOOP('',(#4692,#4693,#4694,#4695)) ;
#1110=EDGE_LOOP('',(#4696,#4697,#4698,#4699)) ;
#1111=EDGE_LOOP('',(#4700,#4701,#4702,#4703)) ;
#1112=EDGE_LOOP('',(#4704,#4705,#4706,#4707)) ;
#1113=EDGE_LOOP('',(#4708,#4709,#4710,#4711)) ;
#1397=LINE('',#9454,#1780) ;
#1398=LINE('',#9469,#1781) ;
#1399=LINE('',#9509,#1782) ;
#1400=LINE('',#9523,#1783) ;
#1401=LINE('',#9543,#1784) ;
#1402=LINE('',#9557,#1785) ;
#1403=LINE('',#9604,#1786) ;
#1404=LINE('',#9606,#1787) ;
#1405=LINE('',#9638,#1788) ;
#1406=LINE('',#9665,#1789) ;
#1407=LINE('',#9712,#1790) ;
#1408=LINE('',#9730,#1791) ;
#1409=LINE('',#9734,#1792) ;
#1410=LINE('',#9762,#1793) ;
#1411=LINE('',#9862,#1794) ;
#1412=LINE('',#9863,#1795) ;
#1413=LINE('',#9865,#1796) ;
#1414=LINE('',#9866,#1797) ;
#1415=LINE('',#9869,#1798) ;
#1416=LINE('',#9871,#1799) ;
#1417=LINE('',#9934,#1800) ;
#1418=LINE('',#9935,#1801) ;
#1419=LINE('',#9943,#1802) ;
#1420=LINE('',#9944,#1803) ;
#1421=LINE('',#9966,#1804) ;
#1422=LINE('',#9968,#1805) ;
#1423=LINE('',#10004,#1806) ;
#1424=LINE('',#10006,#1807) ;
#1425=LINE('',#10024,#1808) ;
#1426=LINE('',#10027,#1809) ;
#1427=LINE('',#10030,#1810) ;
#1428=LINE('',#10031,#1811) ;
#1429=LINE('',#10034,#1812) ;
#1430=LINE('',#10038,#1813) ;
#1431=LINE('',#10039,#1814) ;
#1432=LINE('',#10042,#1815) ;
#1433=LINE('',#10046,#1816) ;
#1434=LINE('',#10047,#1817) ;
#1435=LINE('',#10050,#1818) ;
#1436=LINE('',#10054,#1819) ;
#1437=LINE('',#10058,#1820) ;
#1438=LINE('',#10059,#1821) ;
#1439=LINE('',#10062,#1822) ;
#1440=LINE('',#10066,#1823) ;
#1441=LINE('',#10067,#1824) ;
#1442=LINE('',#10070,#1825) ;
#1443=LINE('',#10074,#1826) ;
#1444=LINE('',#10078,#1827) ;
#1445=LINE('',#10079,#1828) ;
#1446=LINE('',#10082,#1829) ;
#1447=LINE('',#10087,#1830) ;
#1448=LINE('',#10091,#1831) ;
#1449=LINE('',#10125,#1832) ;
#1450=LINE('',#10141,#1833) ;
#1451=LINE('',#10161,#1834) ;
#1452=LINE('',#10175,#1835) ;
#1453=LINE('',#10221,#1836) ;
#1454=LINE('',#10269,#1837) ;
#1455=LINE('',#10271,#1838) ;
#1456=LINE('',#10333,#1839) ;
#1457=LINE('',#10336,#1840) ;
#1458=LINE('',#10395,#1841) ;
#1459=LINE('',#10396,#1842) ;
#1460=LINE('',#10399,#1843) ;
#1461=LINE('',#10458,#1844) ;
#1462=LINE('',#10459,#1845) ;
#1463=LINE('',#10476,#1846) ;
#1464=LINE('',#10505,#1847) ;
#1465=LINE('',#10506,#1848) ;
#1466=LINE('',#10524,#1849) ;
#1467=LINE('',#10538,#1850) ;
#1468=LINE('',#10559,#1851) ;
#1469=LINE('',#10589,#1852) ;
#1470=LINE('',#10626,#1853) ;
#1471=LINE('',#10628,#1854) ;
#1472=LINE('',#10630,#1855) ;
#1473=LINE('',#10632,#1856) ;
#1474=LINE('',#10634,#1857) ;
#1475=LINE('',#10636,#1858) ;
#1476=LINE('',#10638,#1859) ;
#1477=LINE('',#10640,#1860) ;
#1478=LINE('',#10642,#1861) ;
#1479=LINE('',#10644,#1862) ;
#1480=LINE('',#10646,#1863) ;
#1481=LINE('',#10648,#1864) ;
#1482=LINE('',#10650,#1865) ;
#1483=LINE('',#10652,#1866) ;
#1484=LINE('',#10659,#1867) ;
#1485=LINE('',#10662,#1868) ;
#1486=LINE('',#10680,#1869) ;
#1487=LINE('',#10722,#1870) ;
#1488=LINE('',#10727,#1871) ;
#1489=LINE('',#10730,#1872) ;
#1490=LINE('',#10733,#1873) ;
#1491=LINE('',#10734,#1874) ;
#1492=LINE('',#10788,#1875) ;
#1493=LINE('',#10791,#1876) ;
#1494=LINE('',#10793,#1877) ;
#1780=VECTOR('',#7171,10.) ;
#1781=VECTOR('',#7172,10.) ;
#1782=VECTOR('',#7179,10.) ;
#1783=VECTOR('',#7180,10.) ;
#1784=VECTOR('',#7189,10.) ;
#1785=VECTOR('',#7190,10.) ;
#1786=VECTOR('',#7199,10.) ;
#1787=VECTOR('',#7200,10.) ;
#1788=VECTOR('',#7209,10.) ;
#1789=VECTOR('',#7210,10.) ;
#1790=VECTOR('',#7219,10.) ;
#1791=VECTOR('',#7220,10.) ;
#1792=VECTOR('',#7223,10.) ;
#1793=VECTOR('',#7224,10.) ;
#1794=VECTOR('',#7255,10.) ;
#1795=VECTOR('',#7256,10.) ;
#1796=VECTOR('',#7259,10.) ;
#1797=VECTOR('',#7260,10.) ;
#1798=VECTOR('',#7263,10.) ;
#1799=VECTOR('',#7264,10.) ;
#1800=VECTOR('',#7279,10.) ;
#1801=VECTOR('',#7280,10.) ;
#1802=VECTOR('',#7291,10.) ;
#1803=VECTOR('',#7292,10.) ;
#1804=VECTOR('',#7301,10.) ;
#1805=VECTOR('',#7302,10.) ;
#1806=VECTOR('',#7311,10.) ;
#1807=VECTOR('',#7312,10.) ;
#1808=VECTOR('',#7321,10.) ;
#1809=VECTOR('',#7324,10.) ;
#1810=VECTOR('',#7327,10.) ;
#1811=VECTOR('',#7328,10.) ;
#1812=VECTOR('',#7331,10.) ;
#1813=VECTOR('',#7336,10.) ;
#1814=VECTOR('',#7337,10.) ;
#1815=VECTOR('',#7340,10.) ;
#1816=VECTOR('',#7345,10.) ;
#1817=VECTOR('',#7346,10.) ;
#1818=VECTOR('',#7349,10.) ;
#1819=VECTOR('',#7354,10.) ;
#1820=VECTOR('',#7359,10.) ;
#1821=VECTOR('',#7360,10.) ;
#1822=VECTOR('',#7363,10.) ;
#1823=VECTOR('',#7368,10.) ;
#1824=VECTOR('',#7369,10.) ;
#1825=VECTOR('',#7372,10.) ;
#1826=VECTOR('',#7377,10.) ;
#1827=VECTOR('',#7382,10.) ;
#1828=VECTOR('',#7383,10.) ;
#1829=VECTOR('',#7386,10.) ;
#1830=VECTOR('',#7391,10.) ;
#1831=VECTOR('',#7394,10.) ;
#1832=VECTOR('',#7405,10.) ;
#1833=VECTOR('',#7406,10.) ;
#1834=VECTOR('',#7415,10.) ;
#1835=VECTOR('',#7416,10.) ;
#1836=VECTOR('',#7425,10.) ;
#1837=VECTOR('',#7436,10.) ;
#1838=VECTOR('',#7437,10.) ;
#1839=VECTOR('',#7450,10.) ;
#1840=VECTOR('',#7453,10.) ;
#1841=VECTOR('',#7462,10.) ;
#1842=VECTOR('',#7463,10.) ;
#1843=VECTOR('',#7466,10.) ;
#1844=VECTOR('',#7479,10.) ;
#1845=VECTOR('',#7480,10.) ;
#1846=VECTOR('',#7487,10.) ;
#1847=VECTOR('',#7490,10.) ;
#1848=VECTOR('',#7491,10.) ;
#1849=VECTOR('',#7498,10.) ;
#1850=VECTOR('',#7499,10.) ;
#1851=VECTOR('',#7512,10.) ;
#1852=VECTOR('',#7519,10.) ;
#1853=VECTOR('',#7524,10.) ;
#1854=VECTOR('',#7527,10.) ;
#1855=VECTOR('',#7530,10.) ;
#1856=VECTOR('',#7533,10.) ;
#1857=VECTOR('',#7536,10.) ;
#1858=VECTOR('',#7539,10.) ;
#1859=VECTOR('',#7542,10.) ;
#1860=VECTOR('',#7545,10.) ;
#1861=VECTOR('',#7548,10.) ;
#1862=VECTOR('',#7551,10.) ;
#1863=VECTOR('',#7554,10.) ;
#1864=VECTOR('',#7557,10.) ;
#1865=VECTOR('',#7560,10.) ;
#1866=VECTOR('',#7563,10.) ;
#1867=VECTOR('',#7570,10.) ;
#1868=VECTOR('',#7573,10.) ;
#1869=VECTOR('',#7578,10.) ;
#1870=VECTOR('',#7585,10.) ;
#1871=VECTOR('',#7592,10.) ;
#1872=VECTOR('',#7595,10.) ;
#1873=VECTOR('',#7598,10.) ;
#1874=VECTOR('',#7599,10.) ;
#1875=VECTOR('',#7608,10.) ;
#1876=VECTOR('',#7613,3.97) ;
#1877=VECTOR('',#7616,10.) ;
#2120=CIRCLE('',#6040,0.132505429325631) ;
#2121=CIRCLE('',#6041,0.332505429325631) ;
#2122=CIRCLE('',#6044,5.6095419988581) ;
#2123=CIRCLE('',#6045,5.4095419988581) ;
#2124=CIRCLE('',#6048,18.7717409779691) ;
#2125=CIRCLE('',#6049,18.9717409779691) ;
#2126=CIRCLE('',#6052,6.02789861439302) ;
#2127=CIRCLE('',#6053,6.22789861439302) ;
#2128=CIRCLE('',#6056,0.524935224963979) ;
#2129=CIRCLE('',#6057,0.324935224963979) ;
#2130=CIRCLE('',#6062,1.8962519345458) ;
#2131=CIRCLE('',#6063,1.6962519345458) ;
#2132=CIRCLE('',#6065,20.767808830506) ;
#2133=CIRCLE('',#6066,20.567808830506) ;
#2134=CIRCLE('',#6068,6.24675996480777) ;
#2135=CIRCLE('',#6069,6.44675996480776) ;
#2136=CIRCLE('',#6071,9.77267576253889) ;
#2137=CIRCLE('',#6072,0.2) ;
#2138=CIRCLE('',#6073,9.57267576253889) ;
#2139=CIRCLE('',#6078,1.00004201680672) ;
#2140=CIRCLE('',#6079,1.20004201680672) ;
#2141=CIRCLE('',#6081,4.43606098801213) ;
#2142=CIRCLE('',#6082,4.23606098801213) ;
#2143=CIRCLE('',#6085,7.93937148944777) ;
#2144=CIRCLE('',#6086,0.199999999999997) ;
#2145=CIRCLE('',#6087,8.13937148944777) ;
#2146=CIRCLE('',#6090,3.76067266925812) ;
#2147=CIRCLE('',#6091,3.96067266925812) ;
#2148=CIRCLE('',#6094,4.37909654020415) ;
#2149=CIRCLE('',#6095,4.17909654020415) ;
#2150=CIRCLE('',#6098,0.474381812079108) ;
#2151=CIRCLE('',#6099,0.274381812079108) ;
#2152=CIRCLE('',#6101,0.474381812079108) ;
#2153=CIRCLE('',#6104,0.332505429325631) ;
#2154=CIRCLE('',#6107,5.4095419988581) ;
#2155=CIRCLE('',#6110,6.22789861439302) ;
#2156=CIRCLE('',#6112,0.324935224963979) ;
#2157=CIRCLE('',#6115,1.20004201680672) ;
#2158=CIRCLE('',#6118,1.6962519345458) ;
#2159=CIRCLE('',#6120,6.44675996480776) ;
#2160=CIRCLE('',#6123,9.57267576253889) ;
#2161=CIRCLE('',#6125,0.85017716535433) ;
#2162=CIRCLE('',#6126,0.85017716535433) ;
#2163=CIRCLE('',#6127,3.97) ;
#2164=CIRCLE('',#6129,0.274381812079108) ;
#2165=CIRCLE('',#6132,4.37909654020415) ;
#2166=CIRCLE('',#6133,4.17909654020415) ;
#2167=CIRCLE('',#6136,3.96067266925812) ;
#2168=CIRCLE('',#6137,3.76067266925812) ;
#2169=CIRCLE('',#6140,8.13937148944777) ;
#2170=CIRCLE('',#6141,0.2) ;
#2171=CIRCLE('',#6142,7.93937148944777) ;
#2172=CIRCLE('',#6145,1.00004201680672) ;
#2173=CIRCLE('',#6147,4.23606098801213) ;
#2174=CIRCLE('',#6148,4.43606098801213) ;
#2175=CIRCLE('',#6152,0.2) ;
#2176=CIRCLE('',#6153,9.77267576253889) ;
#2177=CIRCLE('',#6157,20.567808830506) ;
#2178=CIRCLE('',#6158,20.767808830506) ;
#2179=CIRCLE('',#6160,6.24675996480777) ;
#2180=CIRCLE('',#6163,1.8962519345458) ;
#2181=CIRCLE('',#6167,0.524935224963979) ;
#2182=CIRCLE('',#6170,18.9717409779691) ;
#2183=CIRCLE('',#6171,18.7717409779691) ;
#2184=CIRCLE('',#6173,6.02789861439302) ;
#2185=CIRCLE('',#6176,5.6095419988581) ;
#2186=CIRCLE('',#6178,0.132505429325631) ;
#2187=CIRCLE('',#6195,0.85017716535433) ;
#2188=CIRCLE('',#6196,0.85017716535433) ;
#2189=CIRCLE('',#6197,3.97) ;
#2190=CIRCLE('',#6200,0.65017716535433) ;
#2191=CIRCLE('',#6203,0.65017716535433) ;
#2192=CIRCLE('',#6205,0.65017716535433) ;
#2193=CIRCLE('',#6208,0.65017716535433) ;
#2489=VERTEX_POINT('',#9452) ;
#2490=VERTEX_POINT('',#9453) ;
#2491=VERTEX_POINT('',#9455) ;
#2492=VERTEX_POINT('',#9468) ;
#2493=VERTEX_POINT('',#9491) ;
#2494=VERTEX_POINT('',#9493) ;
#2495=VERTEX_POINT('',#9508) ;
#2496=VERTEX_POINT('',#9510) ;
#2497=VERTEX_POINT('',#9525) ;
#2498=VERTEX_POINT('',#9527) ;
#2499=VERTEX_POINT('',#9542) ;
#2500=VERTEX_POINT('',#9544) ;
#2501=VERTEX_POINT('',#9559) ;
#2502=VERTEX_POINT('',#9560) ;
#2503=VERTEX_POINT('',#9586) ;
#2504=VERTEX_POINT('',#9588) ;
#2505=VERTEX_POINT('',#9603) ;
#2506=VERTEX_POINT('',#9605) ;
#2507=VERTEX_POINT('',#9620) ;
#2508=VERTEX_POINT('',#9622) ;
#2509=VERTEX_POINT('',#9637) ;
#2510=VERTEX_POINT('',#9639) ;
#2511=VERTEX_POINT('',#9667) ;
#2512=VERTEX_POINT('',#9669) ;
#2513=VERTEX_POINT('',#9684) ;
#2514=VERTEX_POINT('',#9685) ;
#2515=VERTEX_POINT('',#9711) ;
#2516=VERTEX_POINT('',#9713) ;
#2517=VERTEX_POINT('',#9732) ;
#2518=VERTEX_POINT('',#9733) ;
#2519=VERTEX_POINT('',#9735) ;
#2520=VERTEX_POINT('',#9761) ;
#2521=VERTEX_POINT('',#9765) ;
#2522=VERTEX_POINT('',#9767) ;
#2523=VERTEX_POINT('',#9782) ;
#2524=VERTEX_POINT('',#9784) ;
#2525=VERTEX_POINT('',#9812) ;
#2526=VERTEX_POINT('',#9814) ;
#2527=VERTEX_POINT('',#9829) ;
#2528=VERTEX_POINT('',#9830) ;
#2529=VERTEX_POINT('',#9856) ;
#2530=VERTEX_POINT('',#9858) ;
#2531=VERTEX_POINT('',#9868) ;
#2532=VERTEX_POINT('',#9870) ;
#2533=VERTEX_POINT('',#9885) ;
#2534=VERTEX_POINT('',#9886) ;
#2535=VERTEX_POINT('',#9915) ;
#2536=VERTEX_POINT('',#9917) ;
#2537=VERTEX_POINT('',#9937) ;
#2538=VERTEX_POINT('',#9939) ;
#2539=VERTEX_POINT('',#9946) ;
#2540=VERTEX_POINT('',#9948) ;
#2541=VERTEX_POINT('',#9965) ;
#2542=VERTEX_POINT('',#9967) ;
#2543=VERTEX_POINT('',#9984) ;
#2544=VERTEX_POINT('',#9986) ;
#2545=VERTEX_POINT('',#10003) ;
#2546=VERTEX_POINT('',#10005) ;
#2547=VERTEX_POINT('',#10023) ;
#2548=VERTEX_POINT('',#10025) ;
#2549=VERTEX_POINT('',#10029) ;
#2550=VERTEX_POINT('',#10033) ;
#2551=VERTEX_POINT('',#10037) ;
#2552=VERTEX_POINT('',#10041) ;
#2553=VERTEX_POINT('',#10045) ;
#2554=VERTEX_POINT('',#10049) ;
#2555=VERTEX_POINT('',#10053) ;
#2556=VERTEX_POINT('',#10057) ;
#2557=VERTEX_POINT('',#10061) ;
#2558=VERTEX_POINT('',#10065) ;
#2559=VERTEX_POINT('',#10069) ;
#2560=VERTEX_POINT('',#10073) ;
#2561=VERTEX_POINT('',#10077) ;
#2562=VERTEX_POINT('',#10081) ;
#2563=VERTEX_POINT('',#10085) ;
#2564=VERTEX_POINT('',#10086) ;
#2565=VERTEX_POINT('',#10088) ;
#2566=VERTEX_POINT('',#10090) ;
#2567=VERTEX_POINT('',#10093) ;
#2568=VERTEX_POINT('',#10096) ;
#2569=VERTEX_POINT('',#10097) ;
#2570=VERTEX_POINT('',#10124) ;
#2571=VERTEX_POINT('',#10126) ;
#2572=VERTEX_POINT('',#10143) ;
#2573=VERTEX_POINT('',#10145) ;
#2574=VERTEX_POINT('',#10160) ;
#2575=VERTEX_POINT('',#10162) ;
#2576=VERTEX_POINT('',#10177) ;
#2577=VERTEX_POINT('',#10179) ;
#2578=VERTEX_POINT('',#10194) ;
#2579=VERTEX_POINT('',#10220) ;
#2580=VERTEX_POINT('',#10235) ;
#2581=VERTEX_POINT('',#10236) ;
#2582=VERTEX_POINT('',#10262) ;
#2583=VERTEX_POINT('',#10264) ;
#2584=VERTEX_POINT('',#10268) ;
#2585=VERTEX_POINT('',#10270) ;
#2586=VERTEX_POINT('',#10287) ;
#2587=VERTEX_POINT('',#10315) ;
#2588=VERTEX_POINT('',#10317) ;
#2589=VERTEX_POINT('',#10332) ;
#2590=VERTEX_POINT('',#10334) ;
#2591=VERTEX_POINT('',#10338) ;
#2592=VERTEX_POINT('',#10364) ;
#2593=VERTEX_POINT('',#10368) ;
#2594=VERTEX_POINT('',#10369) ;
#2595=VERTEX_POINT('',#10398) ;
#2596=VERTEX_POINT('',#10413) ;
#2597=VERTEX_POINT('',#10414) ;
#2598=VERTEX_POINT('',#10443) ;
#2599=VERTEX_POINT('',#10461) ;
#2600=VERTEX_POINT('',#10478) ;
#2601=VERTEX_POINT('',#10479) ;
#2602=VERTEX_POINT('',#10508) ;
#2603=VERTEX_POINT('',#10523) ;
#2604=VERTEX_POINT('',#10525) ;
#2605=VERTEX_POINT('',#10543) ;
#2606=VERTEX_POINT('',#10558) ;
#2607=VERTEX_POINT('',#10573) ;
#2608=VERTEX_POINT('',#10588) ;
#2609=VERTEX_POINT('',#10611) ;
#2610=VERTEX_POINT('',#10655) ;
#2611=VERTEX_POINT('',#10656) ;
#2612=VERTEX_POINT('',#10658) ;
#2613=VERTEX_POINT('',#10660) ;
#2614=VERTEX_POINT('',#10663) ;
#2615=VERTEX_POINT('',#10666) ;
#2616=VERTEX_POINT('',#10679) ;
#2617=VERTEX_POINT('',#10694) ;
#2618=VERTEX_POINT('',#10709) ;
#2619=VERTEX_POINT('',#10726) ;
#2620=VERTEX_POINT('',#10728) ;
#2621=VERTEX_POINT('',#10732) ;
#2622=VERTEX_POINT('',#10736) ;
#3104=EDGE_CURVE('',#2489,#2490,#1397,.T.) ;
#3105=EDGE_CURVE('',#2490,#2491,#271,.T.) ;
#3106=EDGE_CURVE('',#2491,#2492,#1398,.T.) ;
#3107=EDGE_CURVE('',#2489,#2492,#272,.T.) ;
#3108=EDGE_CURVE('',#2490,#2493,#2120,.T.) ;
#3109=EDGE_CURVE('',#2493,#2494,#273,.T.) ;
#3110=EDGE_CURVE('',#2494,#2491,#2121,.T.) ;
#3111=EDGE_CURVE('',#2493,#2495,#1399,.T.) ;
#3112=EDGE_CURVE('',#2495,#2496,#274,.T.) ;
#3113=EDGE_CURVE('',#2496,#2494,#1400,.T.) ;
#3114=EDGE_CURVE('',#2495,#2497,#2122,.T.) ;
#3115=EDGE_CURVE('',#2497,#2498,#275,.T.) ;
#3116=EDGE_CURVE('',#2498,#2496,#2123,.T.) ;
#3117=EDGE_CURVE('',#2497,#2499,#1401,.T.) ;
#3118=EDGE_CURVE('',#2499,#2500,#276,.T.) ;
#3119=EDGE_CURVE('',#2500,#2498,#1402,.T.) ;
#3120=EDGE_CURVE('',#2501,#2502,#277,.T.) ;
#3121=EDGE_CURVE('',#2502,#2503,#2124,.T.) ;
#3122=EDGE_CURVE('',#2503,#2504,#278,.T.) ;
#3123=EDGE_CURVE('',#2504,#2501,#2125,.T.) ;
#3124=EDGE_CURVE('',#2505,#2504,#1403,.T.) ;
#3125=EDGE_CURVE('',#2503,#2506,#1404,.T.) ;
#3126=EDGE_CURVE('',#2506,#2505,#279,.T.) ;
#3127=EDGE_CURVE('',#2499,#2507,#2126,.T.) ;
#3128=EDGE_CURVE('',#2507,#2508,#280,.T.) ;
#3129=EDGE_CURVE('',#2508,#2500,#2127,.T.) ;
#3130=EDGE_CURVE('',#2501,#2509,#1405,.T.) ;
#3131=EDGE_CURVE('',#2509,#2510,#281,.T.) ;
#3132=EDGE_CURVE('',#2510,#2502,#1406,.T.) ;
#3133=EDGE_CURVE('',#2507,#2511,#2128,.T.) ;
#3134=EDGE_CURVE('',#2511,#2512,#282,.T.) ;
#3135=EDGE_CURVE('',#2512,#2508,#2129,.T.) ;
#3136=EDGE_CURVE('',#2513,#2514,#283,.T.) ;
#3137=EDGE_CURVE('',#2514,#2515,#1407,.T.) ;
#3138=EDGE_CURVE('',#2515,#2516,#284,.T.) ;
#3139=EDGE_CURVE('',#2516,#2513,#1408,.T.) ;
#3140=EDGE_CURVE('',#2517,#2518,#1409,.T.) ;
#3141=EDGE_CURVE('',#2518,#2519,#285,.T.) ;
#3142=EDGE_CURVE('',#2519,#2520,#1410,.T.) ;
#3143=EDGE_CURVE('',#2520,#2517,#394,.T.) ;
#3144=EDGE_CURVE('',#2515,#2521,#2130,.T.) ;
#3145=EDGE_CURVE('',#2521,#2522,#286,.T.) ;
#3146=EDGE_CURVE('',#2522,#2516,#2131,.T.) ;
#3147=EDGE_CURVE('',#2518,#2523,#2132,.T.) ;
#3148=EDGE_CURVE('',#2523,#2524,#287,.T.) ;
#3149=EDGE_CURVE('',#2524,#2519,#2133,.T.) ;
#3150=EDGE_CURVE('',#2521,#2525,#2134,.T.) ;
#3151=EDGE_CURVE('',#2525,#2526,#288,.T.) ;
#3152=EDGE_CURVE('',#2526,#2522,#2135,.T.) ;
#3153=EDGE_CURVE('',#2527,#2528,#289,.T.) ;
#3154=EDGE_CURVE('',#2528,#2529,#2136,.T.) ;
#3155=EDGE_CURVE('',#2529,#2530,#2137,.T.) ;
#3156=EDGE_CURVE('',#2530,#2527,#2138,.T.) ;
#3157=EDGE_CURVE('',#2525,#2528,#1411,.T.) ;
#3158=EDGE_CURVE('',#2527,#2526,#1412,.T.) ;
#3159=EDGE_CURVE('',#2523,#2530,#1413,.T.) ;
#3160=EDGE_CURVE('',#2529,#2524,#1414,.T.) ;
#3161=EDGE_CURVE('',#2531,#2517,#1415,.T.) ;
#3162=EDGE_CURVE('',#2520,#2532,#1416,.T.) ;
#3163=EDGE_CURVE('',#2532,#2531,#290,.T.) ;
#3164=EDGE_CURVE('',#2533,#2534,#291,.T.) ;
#3165=EDGE_CURVE('',#2534,#2514,#2139,.T.) ;
#3166=EDGE_CURVE('',#2513,#2533,#2140,.T.) ;
#3167=EDGE_CURVE('',#2535,#2531,#2141,.T.) ;
#3168=EDGE_CURVE('',#2532,#2536,#2142,.T.) ;
#3169=EDGE_CURVE('',#2536,#2535,#292,.T.) ;
#3170=EDGE_CURVE('',#2511,#2534,#1417,.T.) ;
#3171=EDGE_CURVE('',#2533,#2512,#1418,.T.) ;
#3172=EDGE_CURVE('',#2509,#2537,#2143,.T.) ;
#3173=EDGE_CURVE('',#2537,#2538,#2144,.T.) ;
#3174=EDGE_CURVE('',#2538,#2510,#2145,.T.) ;
#3175=EDGE_CURVE('',#2536,#2538,#1419,.T.) ;
#3176=EDGE_CURVE('',#2537,#2535,#1420,.T.) ;
#3177=EDGE_CURVE('',#2539,#2505,#2146,.T.) ;
#3178=EDGE_CURVE('',#2506,#2540,#2147,.T.) ;
#3179=EDGE_CURVE('',#2540,#2539,#293,.T.) ;
#3180=EDGE_CURVE('',#2541,#2539,#1421,.T.) ;
#3181=EDGE_CURVE('',#2540,#2542,#1422,.T.) ;
#3182=EDGE_CURVE('',#2542,#2541,#294,.T.) ;
#3183=EDGE_CURVE('',#2542,#2543,#2148,.T.) ;
#3184=EDGE_CURVE('',#2543,#2544,#295,.T.) ;
#3185=EDGE_CURVE('',#2544,#2541,#2149,.T.) ;
#3186=EDGE_CURVE('',#2545,#2544,#1423,.T.) ;
#3187=EDGE_CURVE('',#2543,#2546,#1424,.T.) ;
#3188=EDGE_CURVE('',#2546,#2545,#296,.T.) ;
#3189=EDGE_CURVE('',#2492,#2545,#2150,.T.) ;
#3190=EDGE_CURVE('',#2546,#2489,#2151,.T.) ;
#3191=EDGE_CURVE('',#2547,#2492,#1425,.T.) ;
#3192=EDGE_CURVE('',#2548,#2547,#2152,.T.) ;
#3193=EDGE_CURVE('',#2548,#2545,#1426,.T.) ;
#3194=EDGE_CURVE('',#2549,#2491,#1427,.T.) ;
#3195=EDGE_CURVE('',#2547,#2549,#1428,.T.) ;
#3196=EDGE_CURVE('',#2550,#2494,#1429,.T.) ;
#3197=EDGE_CURVE('',#2549,#2550,#2153,.T.) ;
#3198=EDGE_CURVE('',#2551,#2496,#1430,.T.) ;
#3199=EDGE_CURVE('',#2550,#2551,#1431,.T.) ;
#3200=EDGE_CURVE('',#2552,#2498,#1432,.T.) ;
#3201=EDGE_CURVE('',#2551,#2552,#2154,.T.) ;
#3202=EDGE_CURVE('',#2553,#2500,#1433,.T.) ;
#3203=EDGE_CURVE('',#2552,#2553,#1434,.T.) ;
#3204=EDGE_CURVE('',#2554,#2508,#1435,.T.) ;
#3205=EDGE_CURVE('',#2553,#2554,#2155,.T.) ;
#3206=EDGE_CURVE('',#2555,#2512,#1436,.T.) ;
#3207=EDGE_CURVE('',#2554,#2555,#2156,.T.) ;
#3208=EDGE_CURVE('',#2556,#2533,#1437,.T.) ;
#3209=EDGE_CURVE('',#2555,#2556,#1438,.T.) ;
#3210=EDGE_CURVE('',#2557,#2513,#1439,.T.) ;
#3211=EDGE_CURVE('',#2556,#2557,#2157,.T.) ;
#3212=EDGE_CURVE('',#2558,#2516,#1440,.T.) ;
#3213=EDGE_CURVE('',#2557,#2558,#1441,.T.) ;
#3214=EDGE_CURVE('',#2559,#2522,#1442,.T.) ;
#3215=EDGE_CURVE('',#2558,#2559,#2158,.T.) ;
#3216=EDGE_CURVE('',#2560,#2526,#1443,.T.) ;
#3217=EDGE_CURVE('',#2559,#2560,#2159,.T.) ;
#3218=EDGE_CURVE('',#2561,#2527,#1444,.T.) ;
#3219=EDGE_CURVE('',#2560,#2561,#1445,.T.) ;
#3220=EDGE_CURVE('',#2562,#2530,#1446,.T.) ;
#3221=EDGE_CURVE('',#2561,#2562,#2160,.T.) ;
#3222=EDGE_CURVE('',#2563,#2564,#1447,.T.) ;
#3223=EDGE_CURVE('',#2565,#2563,#2161,.T.) ;
#3224=EDGE_CURVE('',#2566,#2565,#1448,.T.) ;
#3225=EDGE_CURVE('',#2564,#2566,#2162,.T.) ;
#3226=EDGE_CURVE('',#2567,#2567,#2163,.T.) ;
#3227=EDGE_CURVE('',#2568,#2569,#2164,.T.) ;
#3228=EDGE_CURVE('',#2569,#2548,#297,.T.) ;
#3229=EDGE_CURVE('',#2568,#2547,#298,.T.) ;
#3230=EDGE_CURVE('',#2569,#2570,#1449,.T.) ;
#3231=EDGE_CURVE('',#2570,#2571,#299,.T.) ;
#3232=EDGE_CURVE('',#2571,#2548,#1450,.T.) ;
#3233=EDGE_CURVE('',#2570,#2572,#2165,.T.) ;
#3234=EDGE_CURVE('',#2572,#2573,#300,.T.) ;
#3235=EDGE_CURVE('',#2573,#2571,#2166,.T.) ;
#3236=EDGE_CURVE('',#2572,#2574,#1451,.T.) ;
#3237=EDGE_CURVE('',#2574,#2575,#301,.T.) ;
#3238=EDGE_CURVE('',#2575,#2573,#1452,.T.) ;
#3239=EDGE_CURVE('',#2574,#2576,#2167,.T.) ;
#3240=EDGE_CURVE('',#2576,#2577,#302,.T.) ;
#3241=EDGE_CURVE('',#2577,#2575,#2168,.T.) ;
#3242=EDGE_CURVE('',#2556,#2578,#303,.T.) ;
#3243=EDGE_CURVE('',#2578,#2579,#1453,.T.) ;
#3244=EDGE_CURVE('',#2579,#2555,#304,.T.) ;
#3245=EDGE_CURVE('',#2580,#2581,#305,.T.) ;
#3246=EDGE_CURVE('',#2581,#2582,#2169,.T.) ;
#3247=EDGE_CURVE('',#2582,#2583,#2170,.T.) ;
#3248=EDGE_CURVE('',#2583,#2580,#2171,.T.) ;
#3249=EDGE_CURVE('',#2584,#2583,#1454,.T.) ;
#3250=EDGE_CURVE('',#2582,#2585,#1455,.T.) ;
#3251=EDGE_CURVE('',#2585,#2584,#306,.T.) ;
#3252=EDGE_CURVE('',#2557,#2586,#307,.T.) ;
#3253=EDGE_CURVE('',#2586,#2578,#2172,.T.) ;
#3254=EDGE_CURVE('',#2585,#2587,#2173,.T.) ;
#3255=EDGE_CURVE('',#2587,#2588,#308,.T.) ;
#3256=EDGE_CURVE('',#2588,#2584,#2174,.T.) ;
#3257=EDGE_CURVE('',#2587,#2589,#1456,.T.) ;
#3258=EDGE_CURVE('',#2589,#2590,#395,.T.) ;
#3259=EDGE_CURVE('',#2590,#2588,#1457,.T.) ;
#3260=EDGE_CURVE('',#2591,#2561,#309,.T.) ;
#3261=EDGE_CURVE('',#2562,#2592,#2175,.T.) ;
#3262=EDGE_CURVE('',#2592,#2591,#2176,.T.) ;
#3263=EDGE_CURVE('',#2593,#2594,#310,.T.) ;
#3264=EDGE_CURVE('',#2594,#2592,#1458,.T.) ;
#3265=EDGE_CURVE('',#2562,#2593,#1459,.T.) ;
#3266=EDGE_CURVE('',#2591,#2595,#1460,.T.) ;
#3267=EDGE_CURVE('',#2595,#2560,#311,.T.) ;
#3268=EDGE_CURVE('',#2596,#2597,#312,.T.) ;
#3269=EDGE_CURVE('',#2597,#2594,#2177,.T.) ;
#3270=EDGE_CURVE('',#2593,#2596,#2178,.T.) ;
#3271=EDGE_CURVE('',#2595,#2598,#2179,.T.) ;
#3272=EDGE_CURVE('',#2598,#2559,#313,.T.) ;
#3273=EDGE_CURVE('',#2589,#2597,#1461,.T.) ;
#3274=EDGE_CURVE('',#2596,#2590,#1462,.T.) ;
#3275=EDGE_CURVE('',#2598,#2599,#2180,.T.) ;
#3276=EDGE_CURVE('',#2599,#2558,#314,.T.) ;
#3277=EDGE_CURVE('',#2599,#2586,#1463,.T.) ;
#3278=EDGE_CURVE('',#2600,#2601,#315,.T.) ;
#3279=EDGE_CURVE('',#2601,#2581,#1464,.T.) ;
#3280=EDGE_CURVE('',#2580,#2600,#1465,.T.) ;
#3281=EDGE_CURVE('',#2579,#2602,#2181,.T.) ;
#3282=EDGE_CURVE('',#2602,#2554,#316,.T.) ;
#3283=EDGE_CURVE('',#2576,#2603,#1466,.T.) ;
#3284=EDGE_CURVE('',#2603,#2604,#317,.T.) ;
#3285=EDGE_CURVE('',#2604,#2577,#1467,.T.) ;
#3286=EDGE_CURVE('',#2600,#2604,#2182,.T.) ;
#3287=EDGE_CURVE('',#2603,#2601,#2183,.T.) ;
#3288=EDGE_CURVE('',#2602,#2605,#2184,.T.) ;
#3289=EDGE_CURVE('',#2605,#2553,#318,.T.) ;
#3290=EDGE_CURVE('',#2605,#2606,#1468,.T.) ;
#3291=EDGE_CURVE('',#2606,#2552,#319,.T.) ;
#3292=EDGE_CURVE('',#2606,#2607,#2185,.T.) ;
#3293=EDGE_CURVE('',#2607,#2551,#320,.T.) ;
#3294=EDGE_CURVE('',#2607,#2608,#1469,.T.) ;
#3295=EDGE_CURVE('',#2608,#2550,#321,.T.) ;
#3296=EDGE_CURVE('',#2608,#2609,#2186,.T.) ;
#3297=EDGE_CURVE('',#2609,#2549,#322,.T.) ;
#3298=EDGE_CURVE('',#2609,#2568,#1470,.T.) ;
#3299=EDGE_CURVE('',#2571,#2544,#1471,.T.) ;
#3300=EDGE_CURVE('',#2573,#2541,#1472,.T.) ;
#3301=EDGE_CURVE('',#2575,#2539,#1473,.T.) ;
#3302=EDGE_CURVE('',#2577,#2505,#1474,.T.) ;
#3303=EDGE_CURVE('',#2604,#2504,#1475,.T.) ;
#3304=EDGE_CURVE('',#2600,#2501,#1476,.T.) ;
#3305=EDGE_CURVE('',#2580,#2509,#1477,.T.) ;
#3306=EDGE_CURVE('',#2583,#2537,#1478,.T.) ;
#3307=EDGE_CURVE('',#2584,#2535,#1479,.T.) ;
#3308=EDGE_CURVE('',#2588,#2531,#1480,.T.) ;
#3309=EDGE_CURVE('',#2590,#2517,#1481,.T.) ;
#3310=EDGE_CURVE('',#2596,#2518,#1482,.T.) ;
#3311=EDGE_CURVE('',#2593,#2523,#1483,.T.) ;
#3312=EDGE_CURVE('',#2610,#2611,#2187,.T.) ;
#3313=EDGE_CURVE('',#2612,#2610,#1484,.T.) ;
#3314=EDGE_CURVE('',#2613,#2612,#2188,.T.) ;
#3315=EDGE_CURVE('',#2611,#2613,#1485,.T.) ;
#3316=EDGE_CURVE('',#2614,#2614,#2189,.T.) ;
#3317=EDGE_CURVE('',#2564,#2615,#323,.T.) ;
#3318=EDGE_CURVE('',#2615,#2616,#1486,.T.) ;
#3319=EDGE_CURVE('',#2563,#2616,#324,.T.) ;
#3320=EDGE_CURVE('',#2566,#2617,#325,.T.) ;
#3321=EDGE_CURVE('',#2617,#2615,#2190,.T.) ;
#3322=EDGE_CURVE('',#2565,#2618,#326,.T.) ;
#3323=EDGE_CURVE('',#2618,#2617,#1487,.T.) ;
#3324=EDGE_CURVE('',#2616,#2618,#2191,.T.) ;
#3325=EDGE_CURVE('',#2619,#2616,#1488,.T.) ;
#3326=EDGE_CURVE('',#2620,#2619,#2192,.T.) ;
#3327=EDGE_CURVE('',#2620,#2618,#1489,.T.) ;
#3328=EDGE_CURVE('',#2621,#2615,#1490,.T.) ;
#3329=EDGE_CURVE('',#2619,#2621,#1491,.T.) ;
#3330=EDGE_CURVE('',#2621,#2622,#2193,.T.) ;
#3331=EDGE_CURVE('',#2622,#2613,#327,.T.) ;
#3332=EDGE_CURVE('',#2612,#2621,#328,.T.) ;
#3333=EDGE_CURVE('',#2611,#2620,#329,.T.) ;
#3334=EDGE_CURVE('',#2610,#2619,#330,.T.) ;
#3335=EDGE_CURVE('',#2622,#2620,#1492,.T.) ;
#3336=EDGE_CURVE('',#2567,#2614,#1493,.T.) ;
#3337=EDGE_CURVE('',#2622,#2617,#1494,.T.) ;
#4244=ORIENTED_EDGE('',*,*,#3104,.T.) ;
#4245=ORIENTED_EDGE('',*,*,#3105,.T.) ;
#4246=ORIENTED_EDGE('',*,*,#3106,.T.) ;
#4247=ORIENTED_EDGE('',*,*,#3107,.F.) ;
#4248=ORIENTED_EDGE('',*,*,#3108,.T.) ;
#4249=ORIENTED_EDGE('',*,*,#3109,.T.) ;
#4250=ORIENTED_EDGE('',*,*,#3110,.T.) ;
#4251=ORIENTED_EDGE('',*,*,#3105,.F.) ;
#4252=ORIENTED_EDGE('',*,*,#3111,.T.) ;
#4253=ORIENTED_EDGE('',*,*,#3112,.T.) ;
#4254=ORIENTED_EDGE('',*,*,#3113,.T.) ;
#4255=ORIENTED_EDGE('',*,*,#3109,.F.) ;
#4256=ORIENTED_EDGE('',*,*,#3114,.T.) ;
#4257=ORIENTED_EDGE('',*,*,#3115,.T.) ;
#4258=ORIENTED_EDGE('',*,*,#3116,.T.) ;
#4259=ORIENTED_EDGE('',*,*,#3112,.F.) ;
#4260=ORIENTED_EDGE('',*,*,#3117,.T.) ;
#4261=ORIENTED_EDGE('',*,*,#3118,.T.) ;
#4262=ORIENTED_EDGE('',*,*,#3119,.T.) ;
#4263=ORIENTED_EDGE('',*,*,#3115,.F.) ;
#4264=ORIENTED_EDGE('',*,*,#3120,.T.) ;
#4265=ORIENTED_EDGE('',*,*,#3121,.T.) ;
#4266=ORIENTED_EDGE('',*,*,#3122,.T.) ;
#4267=ORIENTED_EDGE('',*,*,#3123,.T.) ;
#4268=ORIENTED_EDGE('',*,*,#3124,.T.) ;
#4269=ORIENTED_EDGE('',*,*,#3122,.F.) ;
#4270=ORIENTED_EDGE('',*,*,#3125,.T.) ;
#4271=ORIENTED_EDGE('',*,*,#3126,.T.) ;
#4272=ORIENTED_EDGE('',*,*,#3127,.T.) ;
#4273=ORIENTED_EDGE('',*,*,#3128,.T.) ;
#4274=ORIENTED_EDGE('',*,*,#3129,.T.) ;
#4275=ORIENTED_EDGE('',*,*,#3118,.F.) ;
#4276=ORIENTED_EDGE('',*,*,#3120,.F.) ;
#4277=ORIENTED_EDGE('',*,*,#3130,.T.) ;
#4278=ORIENTED_EDGE('',*,*,#3131,.T.) ;
#4279=ORIENTED_EDGE('',*,*,#3132,.T.) ;
#4280=ORIENTED_EDGE('',*,*,#3133,.T.) ;
#4281=ORIENTED_EDGE('',*,*,#3134,.T.) ;
#4282=ORIENTED_EDGE('',*,*,#3135,.T.) ;
#4283=ORIENTED_EDGE('',*,*,#3128,.F.) ;
#4284=ORIENTED_EDGE('',*,*,#3136,.T.) ;
#4285=ORIENTED_EDGE('',*,*,#3137,.T.) ;
#4286=ORIENTED_EDGE('',*,*,#3138,.T.) ;
#4287=ORIENTED_EDGE('',*,*,#3139,.T.) ;
#4288=ORIENTED_EDGE('',*,*,#3140,.T.) ;
#4289=ORIENTED_EDGE('',*,*,#3141,.T.) ;
#4290=ORIENTED_EDGE('',*,*,#3142,.T.) ;
#4291=ORIENTED_EDGE('',*,*,#3143,.T.) ;
#4292=ORIENTED_EDGE('',*,*,#3144,.T.) ;
#4293=ORIENTED_EDGE('',*,*,#3145,.T.) ;
#4294=ORIENTED_EDGE('',*,*,#3146,.T.) ;
#4295=ORIENTED_EDGE('',*,*,#3138,.F.) ;
#4296=ORIENTED_EDGE('',*,*,#3141,.F.) ;
#4297=ORIENTED_EDGE('',*,*,#3147,.T.) ;
#4298=ORIENTED_EDGE('',*,*,#3148,.T.) ;
#4299=ORIENTED_EDGE('',*,*,#3149,.T.) ;
#4300=ORIENTED_EDGE('',*,*,#3150,.T.) ;
#4301=ORIENTED_EDGE('',*,*,#3151,.T.) ;
#4302=ORIENTED_EDGE('',*,*,#3152,.T.) ;
#4303=ORIENTED_EDGE('',*,*,#3145,.F.) ;
#4304=ORIENTED_EDGE('',*,*,#3153,.T.) ;
#4305=ORIENTED_EDGE('',*,*,#3154,.T.) ;
#4306=ORIENTED_EDGE('',*,*,#3155,.T.) ;
#4307=ORIENTED_EDGE('',*,*,#3156,.T.) ;
#4308=ORIENTED_EDGE('',*,*,#3157,.T.) ;
#4309=ORIENTED_EDGE('',*,*,#3153,.F.) ;
#4310=ORIENTED_EDGE('',*,*,#3158,.T.) ;
#4311=ORIENTED_EDGE('',*,*,#3151,.F.) ;
#4312=ORIENTED_EDGE('',*,*,#3148,.F.) ;
#4313=ORIENTED_EDGE('',*,*,#3159,.T.) ;
#4314=ORIENTED_EDGE('',*,*,#3155,.F.) ;
#4315=ORIENTED_EDGE('',*,*,#3160,.T.) ;
#4316=ORIENTED_EDGE('',*,*,#3161,.T.) ;
#4317=ORIENTED_EDGE('',*,*,#3143,.F.) ;
#4318=ORIENTED_EDGE('',*,*,#3162,.T.) ;
#4319=ORIENTED_EDGE('',*,*,#3163,.T.) ;
#4320=ORIENTED_EDGE('',*,*,#3164,.T.) ;
#4321=ORIENTED_EDGE('',*,*,#3165,.T.) ;
#4322=ORIENTED_EDGE('',*,*,#3136,.F.) ;
#4323=ORIENTED_EDGE('',*,*,#3166,.T.) ;
#4324=ORIENTED_EDGE('',*,*,#3167,.T.) ;
#4325=ORIENTED_EDGE('',*,*,#3163,.F.) ;
#4326=ORIENTED_EDGE('',*,*,#3168,.T.) ;
#4327=ORIENTED_EDGE('',*,*,#3169,.T.) ;
#4328=ORIENTED_EDGE('',*,*,#3170,.T.) ;
#4329=ORIENTED_EDGE('',*,*,#3164,.F.) ;
#4330=ORIENTED_EDGE('',*,*,#3171,.T.) ;
#4331=ORIENTED_EDGE('',*,*,#3134,.F.) ;
#4332=ORIENTED_EDGE('',*,*,#3131,.F.) ;
#4333=ORIENTED_EDGE('',*,*,#3172,.T.) ;
#4334=ORIENTED_EDGE('',*,*,#3173,.T.) ;
#4335=ORIENTED_EDGE('',*,*,#3174,.T.) ;
#4336=ORIENTED_EDGE('',*,*,#3175,.T.) ;
#4337=ORIENTED_EDGE('',*,*,#3173,.F.) ;
#4338=ORIENTED_EDGE('',*,*,#3176,.T.) ;
#4339=ORIENTED_EDGE('',*,*,#3169,.F.) ;
#4340=ORIENTED_EDGE('',*,*,#3177,.T.) ;
#4341=ORIENTED_EDGE('',*,*,#3126,.F.) ;
#4342=ORIENTED_EDGE('',*,*,#3178,.T.) ;
#4343=ORIENTED_EDGE('',*,*,#3179,.T.) ;
#4344=ORIENTED_EDGE('',*,*,#3180,.T.) ;
#4345=ORIENTED_EDGE('',*,*,#3179,.F.) ;
#4346=ORIENTED_EDGE('',*,*,#3181,.T.) ;
#4347=ORIENTED_EDGE('',*,*,#3182,.T.) ;
#4348=ORIENTED_EDGE('',*,*,#3183,.T.) ;
#4349=ORIENTED_EDGE('',*,*,#3184,.T.) ;
#4350=ORIENTED_EDGE('',*,*,#3185,.T.) ;
#4351=ORIENTED_EDGE('',*,*,#3182,.F.) ;
#4352=ORIENTED_EDGE('',*,*,#3186,.T.) ;
#4353=ORIENTED_EDGE('',*,*,#3184,.F.) ;
#4354=ORIENTED_EDGE('',*,*,#3187,.T.) ;
#4355=ORIENTED_EDGE('',*,*,#3188,.T.) ;
#4356=ORIENTED_EDGE('',*,*,#3189,.T.) ;
#4357=ORIENTED_EDGE('',*,*,#3188,.F.) ;
#4358=ORIENTED_EDGE('',*,*,#3190,.T.) ;
#4359=ORIENTED_EDGE('',*,*,#3107,.T.) ;
#4360=ORIENTED_EDGE('',*,*,#3189,.F.) ;
#4361=ORIENTED_EDGE('',*,*,#3191,.F.) ;
#4362=ORIENTED_EDGE('',*,*,#3192,.F.) ;
#4363=ORIENTED_EDGE('',*,*,#3193,.T.) ;
#4364=ORIENTED_EDGE('',*,*,#3106,.F.) ;
#4365=ORIENTED_EDGE('',*,*,#3194,.F.) ;
#4366=ORIENTED_EDGE('',*,*,#3195,.F.) ;
#4367=ORIENTED_EDGE('',*,*,#3191,.T.) ;
#4368=ORIENTED_EDGE('',*,*,#3110,.F.) ;
#4369=ORIENTED_EDGE('',*,*,#3196,.F.) ;
#4370=ORIENTED_EDGE('',*,*,#3197,.F.) ;
#4371=ORIENTED_EDGE('',*,*,#3194,.T.) ;
#4372=ORIENTED_EDGE('',*,*,#3113,.F.) ;
#4373=ORIENTED_EDGE('',*,*,#3198,.F.) ;
#4374=ORIENTED_EDGE('',*,*,#3199,.F.) ;
#4375=ORIENTED_EDGE('',*,*,#3196,.T.) ;
#4376=ORIENTED_EDGE('',*,*,#3116,.F.) ;
#4377=ORIENTED_EDGE('',*,*,#3200,.F.) ;
#4378=ORIENTED_EDGE('',*,*,#3201,.F.) ;
#4379=ORIENTED_EDGE('',*,*,#3198,.T.) ;
#4380=ORIENTED_EDGE('',*,*,#3119,.F.) ;
#4381=ORIENTED_EDGE('',*,*,#3202,.F.) ;
#4382=ORIENTED_EDGE('',*,*,#3203,.F.) ;
#4383=ORIENTED_EDGE('',*,*,#3200,.T.) ;
#4384=ORIENTED_EDGE('',*,*,#3129,.F.) ;
#4385=ORIENTED_EDGE('',*,*,#3204,.F.) ;
#4386=ORIENTED_EDGE('',*,*,#3205,.F.) ;
#4387=ORIENTED_EDGE('',*,*,#3202,.T.) ;
#4388=ORIENTED_EDGE('',*,*,#3135,.F.) ;
#4389=ORIENTED_EDGE('',*,*,#3206,.F.) ;
#4390=ORIENTED_EDGE('',*,*,#3207,.F.) ;
#4391=ORIENTED_EDGE('',*,*,#3204,.T.) ;
#4392=ORIENTED_EDGE('',*,*,#3171,.F.) ;
#4393=ORIENTED_EDGE('',*,*,#3208,.F.) ;
#4394=ORIENTED_EDGE('',*,*,#3209,.F.) ;
#4395=ORIENTED_EDGE('',*,*,#3206,.T.) ;
#4396=ORIENTED_EDGE('',*,*,#3166,.F.) ;
#4397=ORIENTED_EDGE('',*,*,#3210,.F.) ;
#4398=ORIENTED_EDGE('',*,*,#3211,.F.) ;
#4399=ORIENTED_EDGE('',*,*,#3208,.T.) ;
#4400=ORIENTED_EDGE('',*,*,#3139,.F.) ;
#4401=ORIENTED_EDGE('',*,*,#3212,.F.) ;
#4402=ORIENTED_EDGE('',*,*,#3213,.F.) ;
#4403=ORIENTED_EDGE('',*,*,#3210,.T.) ;
#4404=ORIENTED_EDGE('',*,*,#3146,.F.) ;
#4405=ORIENTED_EDGE('',*,*,#3214,.F.) ;
#4406=ORIENTED_EDGE('',*,*,#3215,.F.) ;
#4407=ORIENTED_EDGE('',*,*,#3212,.T.) ;
#4408=ORIENTED_EDGE('',*,*,#3152,.F.) ;
#4409=ORIENTED_EDGE('',*,*,#3216,.F.) ;
#4410=ORIENTED_EDGE('',*,*,#3217,.F.) ;
#4411=ORIENTED_EDGE('',*,*,#3214,.T.) ;
#4412=ORIENTED_EDGE('',*,*,#3158,.F.) ;
#4413=ORIENTED_EDGE('',*,*,#3218,.F.) ;
#4414=ORIENTED_EDGE('',*,*,#3219,.F.) ;
#4415=ORIENTED_EDGE('',*,*,#3216,.T.) ;
#4416=ORIENTED_EDGE('',*,*,#3156,.F.) ;
#4417=ORIENTED_EDGE('',*,*,#3220,.F.) ;
#4418=ORIENTED_EDGE('',*,*,#3221,.F.) ;
#4419=ORIENTED_EDGE('',*,*,#3218,.T.) ;
#4420=ORIENTED_EDGE('',*,*,#3154,.F.) ;
#4421=ORIENTED_EDGE('',*,*,#3157,.F.) ;
#4422=ORIENTED_EDGE('',*,*,#3150,.F.) ;
#4423=ORIENTED_EDGE('',*,*,#3144,.F.) ;
#4424=ORIENTED_EDGE('',*,*,#3137,.F.) ;
#4425=ORIENTED_EDGE('',*,*,#3165,.F.) ;
#4426=ORIENTED_EDGE('',*,*,#3170,.F.) ;
#4427=ORIENTED_EDGE('',*,*,#3133,.F.) ;
#4428=ORIENTED_EDGE('',*,*,#3127,.F.) ;
#4429=ORIENTED_EDGE('',*,*,#3117,.F.) ;
#4430=ORIENTED_EDGE('',*,*,#3114,.F.) ;
#4431=ORIENTED_EDGE('',*,*,#3111,.F.) ;
#4432=ORIENTED_EDGE('',*,*,#3108,.F.) ;
#4433=ORIENTED_EDGE('',*,*,#3104,.F.) ;
#4434=ORIENTED_EDGE('',*,*,#3190,.F.) ;
#4435=ORIENTED_EDGE('',*,*,#3187,.F.) ;
#4436=ORIENTED_EDGE('',*,*,#3183,.F.) ;
#4437=ORIENTED_EDGE('',*,*,#3181,.F.) ;
#4438=ORIENTED_EDGE('',*,*,#3178,.F.) ;
#4439=ORIENTED_EDGE('',*,*,#3125,.F.) ;
#4440=ORIENTED_EDGE('',*,*,#3121,.F.) ;
#4441=ORIENTED_EDGE('',*,*,#3132,.F.) ;
#4442=ORIENTED_EDGE('',*,*,#3174,.F.) ;
#4443=ORIENTED_EDGE('',*,*,#3175,.F.) ;
#4444=ORIENTED_EDGE('',*,*,#3168,.F.) ;
#4445=ORIENTED_EDGE('',*,*,#3162,.F.) ;
#4446=ORIENTED_EDGE('',*,*,#3142,.F.) ;
#4447=ORIENTED_EDGE('',*,*,#3149,.F.) ;
#4448=ORIENTED_EDGE('',*,*,#3160,.F.) ;
#4449=ORIENTED_EDGE('',*,*,#3222,.F.) ;
#4450=ORIENTED_EDGE('',*,*,#3223,.F.) ;
#4451=ORIENTED_EDGE('',*,*,#3224,.F.) ;
#4452=ORIENTED_EDGE('',*,*,#3225,.F.) ;
#4453=ORIENTED_EDGE('',*,*,#3226,.T.) ;
#4454=ORIENTED_EDGE('',*,*,#3227,.T.) ;
#4455=ORIENTED_EDGE('',*,*,#3228,.T.) ;
#4456=ORIENTED_EDGE('',*,*,#3192,.T.) ;
#4457=ORIENTED_EDGE('',*,*,#3229,.F.) ;
#4458=ORIENTED_EDGE('',*,*,#3230,.T.) ;
#4459=ORIENTED_EDGE('',*,*,#3231,.T.) ;
#4460=ORIENTED_EDGE('',*,*,#3232,.T.) ;
#4461=ORIENTED_EDGE('',*,*,#3228,.F.) ;
#4462=ORIENTED_EDGE('',*,*,#3233,.T.) ;
#4463=ORIENTED_EDGE('',*,*,#3234,.T.) ;
#4464=ORIENTED_EDGE('',*,*,#3235,.T.) ;
#4465=ORIENTED_EDGE('',*,*,#3231,.F.) ;
#4466=ORIENTED_EDGE('',*,*,#3236,.T.) ;
#4467=ORIENTED_EDGE('',*,*,#3237,.T.) ;
#4468=ORIENTED_EDGE('',*,*,#3238,.T.) ;
#4469=ORIENTED_EDGE('',*,*,#3234,.F.) ;
#4470=ORIENTED_EDGE('',*,*,#3239,.T.) ;
#4471=ORIENTED_EDGE('',*,*,#3240,.T.) ;
#4472=ORIENTED_EDGE('',*,*,#3241,.T.) ;
#4473=ORIENTED_EDGE('',*,*,#3237,.F.) ;
#4474=ORIENTED_EDGE('',*,*,#3209,.T.) ;
#4475=ORIENTED_EDGE('',*,*,#3242,.T.) ;
#4476=ORIENTED_EDGE('',*,*,#3243,.T.) ;
#4477=ORIENTED_EDGE('',*,*,#3244,.T.) ;
#4478=ORIENTED_EDGE('',*,*,#3245,.T.) ;
#4479=ORIENTED_EDGE('',*,*,#3246,.T.) ;
#4480=ORIENTED_EDGE('',*,*,#3247,.T.) ;
#4481=ORIENTED_EDGE('',*,*,#3248,.T.) ;
#4482=ORIENTED_EDGE('',*,*,#3249,.T.) ;
#4483=ORIENTED_EDGE('',*,*,#3247,.F.) ;
#4484=ORIENTED_EDGE('',*,*,#3250,.T.) ;
#4485=ORIENTED_EDGE('',*,*,#3251,.T.) ;
#4486=ORIENTED_EDGE('',*,*,#3242,.F.) ;
#4487=ORIENTED_EDGE('',*,*,#3211,.T.) ;
#4488=ORIENTED_EDGE('',*,*,#3252,.T.) ;
#4489=ORIENTED_EDGE('',*,*,#3253,.T.) ;
#4490=ORIENTED_EDGE('',*,*,#3254,.T.) ;
#4491=ORIENTED_EDGE('',*,*,#3255,.T.) ;
#4492=ORIENTED_EDGE('',*,*,#3256,.T.) ;
#4493=ORIENTED_EDGE('',*,*,#3251,.F.) ;
#4494=ORIENTED_EDGE('',*,*,#3257,.T.) ;
#4495=ORIENTED_EDGE('',*,*,#3258,.T.) ;
#4496=ORIENTED_EDGE('',*,*,#3259,.T.) ;
#4497=ORIENTED_EDGE('',*,*,#3255,.F.) ;
#4498=ORIENTED_EDGE('',*,*,#3260,.T.) ;
#4499=ORIENTED_EDGE('',*,*,#3221,.T.) ;
#4500=ORIENTED_EDGE('',*,*,#3261,.T.) ;
#4501=ORIENTED_EDGE('',*,*,#3262,.T.) ;
#4502=ORIENTED_EDGE('',*,*,#3263,.T.) ;
#4503=ORIENTED_EDGE('',*,*,#3264,.T.) ;
#4504=ORIENTED_EDGE('',*,*,#3261,.F.) ;
#4505=ORIENTED_EDGE('',*,*,#3265,.T.) ;
#4506=ORIENTED_EDGE('',*,*,#3219,.T.) ;
#4507=ORIENTED_EDGE('',*,*,#3260,.F.) ;
#4508=ORIENTED_EDGE('',*,*,#3266,.T.) ;
#4509=ORIENTED_EDGE('',*,*,#3267,.T.) ;
#4510=ORIENTED_EDGE('',*,*,#3268,.T.) ;
#4511=ORIENTED_EDGE('',*,*,#3269,.T.) ;
#4512=ORIENTED_EDGE('',*,*,#3263,.F.) ;
#4513=ORIENTED_EDGE('',*,*,#3270,.T.) ;
#4514=ORIENTED_EDGE('',*,*,#3217,.T.) ;
#4515=ORIENTED_EDGE('',*,*,#3267,.F.) ;
#4516=ORIENTED_EDGE('',*,*,#3271,.T.) ;
#4517=ORIENTED_EDGE('',*,*,#3272,.T.) ;
#4518=ORIENTED_EDGE('',*,*,#3273,.T.) ;
#4519=ORIENTED_EDGE('',*,*,#3268,.F.) ;
#4520=ORIENTED_EDGE('',*,*,#3274,.T.) ;
#4521=ORIENTED_EDGE('',*,*,#3258,.F.) ;
#4522=ORIENTED_EDGE('',*,*,#3215,.T.) ;
#4523=ORIENTED_EDGE('',*,*,#3272,.F.) ;
#4524=ORIENTED_EDGE('',*,*,#3275,.T.) ;
#4525=ORIENTED_EDGE('',*,*,#3276,.T.) ;
#4526=ORIENTED_EDGE('',*,*,#3252,.F.) ;
#4527=ORIENTED_EDGE('',*,*,#3213,.T.) ;
#4528=ORIENTED_EDGE('',*,*,#3276,.F.) ;
#4529=ORIENTED_EDGE('',*,*,#3277,.T.) ;
#4530=ORIENTED_EDGE('',*,*,#3278,.T.) ;
#4531=ORIENTED_EDGE('',*,*,#3279,.T.) ;
#4532=ORIENTED_EDGE('',*,*,#3245,.F.) ;
#4533=ORIENTED_EDGE('',*,*,#3280,.T.) ;
#4534=ORIENTED_EDGE('',*,*,#3207,.T.) ;
#4535=ORIENTED_EDGE('',*,*,#3244,.F.) ;
#4536=ORIENTED_EDGE('',*,*,#3281,.T.) ;
#4537=ORIENTED_EDGE('',*,*,#3282,.T.) ;
#4538=ORIENTED_EDGE('',*,*,#3283,.T.) ;
#4539=ORIENTED_EDGE('',*,*,#3284,.T.) ;
#4540=ORIENTED_EDGE('',*,*,#3285,.T.) ;
#4541=ORIENTED_EDGE('',*,*,#3240,.F.) ;
#4542=ORIENTED_EDGE('',*,*,#3278,.F.) ;
#4543=ORIENTED_EDGE('',*,*,#3286,.T.) ;
#4544=ORIENTED_EDGE('',*,*,#3284,.F.) ;
#4545=ORIENTED_EDGE('',*,*,#3287,.T.) ;
#4546=ORIENTED_EDGE('',*,*,#3205,.T.) ;
#4547=ORIENTED_EDGE('',*,*,#3282,.F.) ;
#4548=ORIENTED_EDGE('',*,*,#3288,.T.) ;
#4549=ORIENTED_EDGE('',*,*,#3289,.T.) ;
#4550=ORIENTED_EDGE('',*,*,#3203,.T.) ;
#4551=ORIENTED_EDGE('',*,*,#3289,.F.) ;
#4552=ORIENTED_EDGE('',*,*,#3290,.T.) ;
#4553=ORIENTED_EDGE('',*,*,#3291,.T.) ;
#4554=ORIENTED_EDGE('',*,*,#3201,.T.) ;
#4555=ORIENTED_EDGE('',*,*,#3291,.F.) ;
#4556=ORIENTED_EDGE('',*,*,#3292,.T.) ;
#4557=ORIENTED_EDGE('',*,*,#3293,.T.) ;
#4558=ORIENTED_EDGE('',*,*,#3199,.T.) ;
#4559=ORIENTED_EDGE('',*,*,#3293,.F.) ;
#4560=ORIENTED_EDGE('',*,*,#3294,.T.) ;
#4561=ORIENTED_EDGE('',*,*,#3295,.T.) ;
#4562=ORIENTED_EDGE('',*,*,#3197,.T.) ;
#4563=ORIENTED_EDGE('',*,*,#3295,.F.) ;
#4564=ORIENTED_EDGE('',*,*,#3296,.T.) ;
#4565=ORIENTED_EDGE('',*,*,#3297,.T.) ;
#4566=ORIENTED_EDGE('',*,*,#3195,.T.) ;
#4567=ORIENTED_EDGE('',*,*,#3297,.F.) ;
#4568=ORIENTED_EDGE('',*,*,#3298,.T.) ;
#4569=ORIENTED_EDGE('',*,*,#3229,.T.) ;
#4570=ORIENTED_EDGE('',*,*,#3186,.F.) ;
#4571=ORIENTED_EDGE('',*,*,#3193,.F.) ;
#4572=ORIENTED_EDGE('',*,*,#3232,.F.) ;
#4573=ORIENTED_EDGE('',*,*,#3299,.T.) ;
#4574=ORIENTED_EDGE('',*,*,#3185,.F.) ;
#4575=ORIENTED_EDGE('',*,*,#3299,.F.) ;
#4576=ORIENTED_EDGE('',*,*,#3235,.F.) ;
#4577=ORIENTED_EDGE('',*,*,#3300,.T.) ;
#4578=ORIENTED_EDGE('',*,*,#3180,.F.) ;
#4579=ORIENTED_EDGE('',*,*,#3300,.F.) ;
#4580=ORIENTED_EDGE('',*,*,#3238,.F.) ;
#4581=ORIENTED_EDGE('',*,*,#3301,.T.) ;
#4582=ORIENTED_EDGE('',*,*,#3177,.F.) ;
#4583=ORIENTED_EDGE('',*,*,#3301,.F.) ;
#4584=ORIENTED_EDGE('',*,*,#3241,.F.) ;
#4585=ORIENTED_EDGE('',*,*,#3302,.T.) ;
#4586=ORIENTED_EDGE('',*,*,#3124,.F.) ;
#4587=ORIENTED_EDGE('',*,*,#3302,.F.) ;
#4588=ORIENTED_EDGE('',*,*,#3285,.F.) ;
#4589=ORIENTED_EDGE('',*,*,#3303,.T.) ;
#4590=ORIENTED_EDGE('',*,*,#3123,.F.) ;
#4591=ORIENTED_EDGE('',*,*,#3303,.F.) ;
#4592=ORIENTED_EDGE('',*,*,#3286,.F.) ;
#4593=ORIENTED_EDGE('',*,*,#3304,.T.) ;
#4594=ORIENTED_EDGE('',*,*,#3130,.F.) ;
#4595=ORIENTED_EDGE('',*,*,#3304,.F.) ;
#4596=ORIENTED_EDGE('',*,*,#3280,.F.) ;
#4597=ORIENTED_EDGE('',*,*,#3305,.T.) ;
#4598=ORIENTED_EDGE('',*,*,#3172,.F.) ;
#4599=ORIENTED_EDGE('',*,*,#3305,.F.) ;
#4600=ORIENTED_EDGE('',*,*,#3248,.F.) ;
#4601=ORIENTED_EDGE('',*,*,#3306,.T.) ;
#4602=ORIENTED_EDGE('',*,*,#3176,.F.) ;
#4603=ORIENTED_EDGE('',*,*,#3306,.F.) ;
#4604=ORIENTED_EDGE('',*,*,#3249,.F.) ;
#4605=ORIENTED_EDGE('',*,*,#3307,.T.) ;
#4606=ORIENTED_EDGE('',*,*,#3167,.F.) ;
#4607=ORIENTED_EDGE('',*,*,#3307,.F.) ;
#4608=ORIENTED_EDGE('',*,*,#3256,.F.) ;
#4609=ORIENTED_EDGE('',*,*,#3308,.T.) ;
#4610=ORIENTED_EDGE('',*,*,#3161,.F.) ;
#4611=ORIENTED_EDGE('',*,*,#3308,.F.) ;
#4612=ORIENTED_EDGE('',*,*,#3259,.F.) ;
#4613=ORIENTED_EDGE('',*,*,#3309,.T.) ;
#4614=ORIENTED_EDGE('',*,*,#3140,.F.) ;
#4615=ORIENTED_EDGE('',*,*,#3309,.F.) ;
#4616=ORIENTED_EDGE('',*,*,#3274,.F.) ;
#4617=ORIENTED_EDGE('',*,*,#3310,.T.) ;
#4618=ORIENTED_EDGE('',*,*,#3147,.F.) ;
#4619=ORIENTED_EDGE('',*,*,#3310,.F.) ;
#4620=ORIENTED_EDGE('',*,*,#3270,.F.) ;
#4621=ORIENTED_EDGE('',*,*,#3311,.T.) ;
#4622=ORIENTED_EDGE('',*,*,#3159,.F.) ;
#4623=ORIENTED_EDGE('',*,*,#3311,.F.) ;
#4624=ORIENTED_EDGE('',*,*,#3265,.F.) ;
#4625=ORIENTED_EDGE('',*,*,#3220,.T.) ;
#4626=ORIENTED_EDGE('',*,*,#3262,.F.) ;
#4627=ORIENTED_EDGE('',*,*,#3264,.F.) ;
#4628=ORIENTED_EDGE('',*,*,#3269,.F.) ;
#4629=ORIENTED_EDGE('',*,*,#3273,.F.) ;
#4630=ORIENTED_EDGE('',*,*,#3257,.F.) ;
#4631=ORIENTED_EDGE('',*,*,#3254,.F.) ;
#4632=ORIENTED_EDGE('',*,*,#3250,.F.) ;
#4633=ORIENTED_EDGE('',*,*,#3246,.F.) ;
#4634=ORIENTED_EDGE('',*,*,#3279,.F.) ;
#4635=ORIENTED_EDGE('',*,*,#3287,.F.) ;
#4636=ORIENTED_EDGE('',*,*,#3283,.F.) ;
#4637=ORIENTED_EDGE('',*,*,#3239,.F.) ;
#4638=ORIENTED_EDGE('',*,*,#3236,.F.) ;
#4639=ORIENTED_EDGE('',*,*,#3233,.F.) ;
#4640=ORIENTED_EDGE('',*,*,#3230,.F.) ;
#4641=ORIENTED_EDGE('',*,*,#3227,.F.) ;
#4642=ORIENTED_EDGE('',*,*,#3298,.F.) ;
#4643=ORIENTED_EDGE('',*,*,#3296,.F.) ;
#4644=ORIENTED_EDGE('',*,*,#3294,.F.) ;
#4645=ORIENTED_EDGE('',*,*,#3292,.F.) ;
#4646=ORIENTED_EDGE('',*,*,#3290,.F.) ;
#4647=ORIENTED_EDGE('',*,*,#3288,.F.) ;
#4648=ORIENTED_EDGE('',*,*,#3281,.F.) ;
#4649=ORIENTED_EDGE('',*,*,#3243,.F.) ;
#4650=ORIENTED_EDGE('',*,*,#3253,.F.) ;
#4651=ORIENTED_EDGE('',*,*,#3277,.F.) ;
#4652=ORIENTED_EDGE('',*,*,#3275,.F.) ;
#4653=ORIENTED_EDGE('',*,*,#3271,.F.) ;
#4654=ORIENTED_EDGE('',*,*,#3266,.F.) ;
#4655=ORIENTED_EDGE('',*,*,#3312,.F.) ;
#4656=ORIENTED_EDGE('',*,*,#3313,.F.) ;
#4657=ORIENTED_EDGE('',*,*,#3314,.F.) ;
#4658=ORIENTED_EDGE('',*,*,#3315,.F.) ;
#4659=ORIENTED_EDGE('',*,*,#3316,.F.) ;
#4660=ORIENTED_EDGE('',*,*,#3222,.T.) ;
#4661=ORIENTED_EDGE('',*,*,#3317,.T.) ;
#4662=ORIENTED_EDGE('',*,*,#3318,.T.) ;
#4663=ORIENTED_EDGE('',*,*,#3319,.F.) ;
#4664=ORIENTED_EDGE('',*,*,#3225,.T.) ;
#4665=ORIENTED_EDGE('',*,*,#3320,.T.) ;
#4666=ORIENTED_EDGE('',*,*,#3321,.T.) ;
#4667=ORIENTED_EDGE('',*,*,#3317,.F.) ;
#4668=ORIENTED_EDGE('',*,*,#3224,.T.) ;
#4669=ORIENTED_EDGE('',*,*,#3322,.T.) ;
#4670=ORIENTED_EDGE('',*,*,#3323,.T.) ;
#4671=ORIENTED_EDGE('',*,*,#3320,.F.) ;
#4672=ORIENTED_EDGE('',*,*,#3324,.T.) ;
#4673=ORIENTED_EDGE('',*,*,#3322,.F.) ;
#4674=ORIENTED_EDGE('',*,*,#3223,.T.) ;
#4675=ORIENTED_EDGE('',*,*,#3319,.T.) ;
#4676=ORIENTED_EDGE('',*,*,#3324,.F.) ;
#4677=ORIENTED_EDGE('',*,*,#3325,.F.) ;
#4678=ORIENTED_EDGE('',*,*,#3326,.F.) ;
#4679=ORIENTED_EDGE('',*,*,#3327,.T.) ;
#4680=ORIENTED_EDGE('',*,*,#3318,.F.) ;
#4681=ORIENTED_EDGE('',*,*,#3328,.F.) ;
#4682=ORIENTED_EDGE('',*,*,#3329,.F.) ;
#4683=ORIENTED_EDGE('',*,*,#3325,.T.) ;
#4684=ORIENTED_EDGE('',*,*,#3330,.T.) ;
#4685=ORIENTED_EDGE('',*,*,#3331,.T.) ;
#4686=ORIENTED_EDGE('',*,*,#3314,.T.) ;
#4687=ORIENTED_EDGE('',*,*,#3332,.T.) ;
#4688=ORIENTED_EDGE('',*,*,#3312,.T.) ;
#4689=ORIENTED_EDGE('',*,*,#3333,.T.) ;
#4690=ORIENTED_EDGE('',*,*,#3326,.T.) ;
#4691=ORIENTED_EDGE('',*,*,#3334,.F.) ;
#4692=ORIENTED_EDGE('',*,*,#3335,.T.) ;
#4693=ORIENTED_EDGE('',*,*,#3333,.F.) ;
#4694=ORIENTED_EDGE('',*,*,#3315,.T.) ;
#4695=ORIENTED_EDGE('',*,*,#3331,.F.) ;
#4696=ORIENTED_EDGE('',*,*,#3329,.T.) ;
#4697=ORIENTED_EDGE('',*,*,#3332,.F.) ;
#4698=ORIENTED_EDGE('',*,*,#3313,.T.) ;
#4699=ORIENTED_EDGE('',*,*,#3334,.T.) ;
#4700=ORIENTED_EDGE('',*,*,#3226,.F.) ;
#4701=ORIENTED_EDGE('',*,*,#3336,.T.) ;
#4702=ORIENTED_EDGE('',*,*,#3316,.T.) ;
#4703=ORIENTED_EDGE('',*,*,#3336,.F.) ;
#4704=ORIENTED_EDGE('',*,*,#3323,.F.) ;
#4705=ORIENTED_EDGE('',*,*,#3327,.F.) ;
#4706=ORIENTED_EDGE('',*,*,#3335,.F.) ;
#4707=ORIENTED_EDGE('',*,*,#3337,.T.) ;
#4708=ORIENTED_EDGE('',*,*,#3321,.F.) ;
#4709=ORIENTED_EDGE('',*,*,#3337,.F.) ;
#4710=ORIENTED_EDGE('',*,*,#3330,.F.) ;
#4711=ORIENTED_EDGE('',*,*,#3328,.T.) ;
#5154=CYLINDRICAL_SURFACE('',#6039,0.2) ;
#5155=CYLINDRICAL_SURFACE('',#6042,0.2) ;
#5156=CYLINDRICAL_SURFACE('',#6046,0.2) ;
#5157=CYLINDRICAL_SURFACE('',#6050,0.2) ;
#5158=CYLINDRICAL_SURFACE('',#6054,0.2) ;
#5159=CYLINDRICAL_SURFACE('',#6058,0.2) ;
#5160=CYLINDRICAL_SURFACE('',#6059,0.2) ;
#5161=CYLINDRICAL_SURFACE('',#6074,0.2) ;
#5162=CYLINDRICAL_SURFACE('',#6075,0.2) ;
#5163=CYLINDRICAL_SURFACE('',#6076,0.2) ;
#5164=CYLINDRICAL_SURFACE('',#6083,0.2) ;
#5165=CYLINDRICAL_SURFACE('',#6088,0.2) ;
#5166=CYLINDRICAL_SURFACE('',#6092,0.2) ;
#5167=CYLINDRICAL_SURFACE('',#6096,0.2) ;
#5168=CYLINDRICAL_SURFACE('',#6100,0.474381812079108) ;
#5169=CYLINDRICAL_SURFACE('',#6103,0.332505429325631) ;
#5170=CYLINDRICAL_SURFACE('',#6106,5.4095419988581) ;
#5171=CYLINDRICAL_SURFACE('',#6109,6.22789861439302) ;
#5172=CYLINDRICAL_SURFACE('',#6111,0.324935224963979) ;
#5173=CYLINDRICAL_SURFACE('',#6114,1.20004201680672) ;
#5174=CYLINDRICAL_SURFACE('',#6117,1.6962519345458) ;
#5175=CYLINDRICAL_SURFACE('',#6119,6.44675996480777) ;
#5176=CYLINDRICAL_SURFACE('',#6122,9.57267576253889) ;
#5177=CYLINDRICAL_SURFACE('',#6130,0.2) ;
#5178=CYLINDRICAL_SURFACE('',#6134,0.2) ;
#5179=CYLINDRICAL_SURFACE('',#6138,0.2) ;
#5180=CYLINDRICAL_SURFACE('',#6143,0.2) ;
#5181=CYLINDRICAL_SURFACE('',#6149,0.2) ;
#5182=CYLINDRICAL_SURFACE('',#6154,0.2) ;
#5183=CYLINDRICAL_SURFACE('',#6155,0.2) ;
#5184=CYLINDRICAL_SURFACE('',#6161,0.2) ;
#5185=CYLINDRICAL_SURFACE('',#6164,0.2) ;
#5186=CYLINDRICAL_SURFACE('',#6165,0.2) ;
#5187=CYLINDRICAL_SURFACE('',#6168,0.2) ;
#5188=CYLINDRICAL_SURFACE('',#6174,0.2) ;
#5189=CYLINDRICAL_SURFACE('',#6177,0.2) ;
#5190=CYLINDRICAL_SURFACE('',#6179,0.2) ;
#5191=CYLINDRICAL_SURFACE('',#6181,4.17909654020415) ;
#5192=CYLINDRICAL_SURFACE('',#6183,3.76067266925812) ;
#5193=CYLINDRICAL_SURFACE('',#6185,18.9717409779691) ;
#5194=CYLINDRICAL_SURFACE('',#6187,7.93937148944777) ;
#5195=CYLINDRICAL_SURFACE('',#6189,4.43606098801213) ;
#5196=CYLINDRICAL_SURFACE('',#6192,20.767808830506) ;
#5197=CYLINDRICAL_SURFACE('',#6198,0.2) ;
#5198=CYLINDRICAL_SURFACE('',#6201,0.2) ;
#5199=CYLINDRICAL_SURFACE('',#6204,0.65017716535433) ;
#5200=CYLINDRICAL_SURFACE('',#6210,0.2) ;
#5201=CYLINDRICAL_SURFACE('',#6211,0.2) ;
#5202=CYLINDRICAL_SURFACE('',#6212,3.97) ;
#5203=CYLINDRICAL_SURFACE('',#6214,0.65017716535433) ;
#5375=ADVANCED_FACE('',(#650),#5154,.T.) ;
#5376=ADVANCED_FACE('',(#651),#106,.F.) ;
#5377=ADVANCED_FACE('',(#652),#5155,.T.) ;
#5378=ADVANCED_FACE('',(#653),#202,.T.) ;
#5379=ADVANCED_FACE('',(#654),#5156,.T.) ;
#5380=ADVANCED_FACE('',(#655),#203,.T.) ;
#5381=ADVANCED_FACE('',(#656),#5157,.T.) ;
#5382=ADVANCED_FACE('',(#657),#204,.T.) ;
#5383=ADVANCED_FACE('',(#658),#5158,.T.) ;
#5384=ADVANCED_FACE('',(#659),#205,.T.) ;
#5385=ADVANCED_FACE('',(#660),#5159,.T.) ;
#5386=ADVANCED_FACE('',(#661),#5160,.T.) ;
#5387=ADVANCED_FACE('',(#662),#206,.T.) ;
#5388=ADVANCED_FACE('',(#663),#207,.T.) ;
#5389=ADVANCED_FACE('',(#664),#208,.T.) ;
#5390=ADVANCED_FACE('',(#665),#209,.T.) ;
#5391=ADVANCED_FACE('',(#666),#5161,.T.) ;
#5392=ADVANCED_FACE('',(#667),#5162,.T.) ;
#5393=ADVANCED_FACE('',(#668),#5163,.T.) ;
#5394=ADVANCED_FACE('',(#669),#210,.T.) ;
#5395=ADVANCED_FACE('',(#670),#211,.T.) ;
#5396=ADVANCED_FACE('',(#671),#5164,.T.) ;
#5397=ADVANCED_FACE('',(#672),#212,.T.) ;
#5398=ADVANCED_FACE('',(#673),#5165,.T.) ;
#5399=ADVANCED_FACE('',(#674),#213,.T.) ;
#5400=ADVANCED_FACE('',(#675),#5166,.T.) ;
#5401=ADVANCED_FACE('',(#676),#214,.T.) ;
#5402=ADVANCED_FACE('',(#677),#5167,.T.) ;
#5403=ADVANCED_FACE('',(#678),#215,.T.) ;
#5404=ADVANCED_FACE('',(#679),#5168,.T.) ;
#5405=ADVANCED_FACE('',(#680),#442,.T.) ;
#5406=ADVANCED_FACE('',(#681),#5169,.T.) ;
#5407=ADVANCED_FACE('',(#682),#443,.T.) ;
#5408=ADVANCED_FACE('',(#683),#5170,.F.) ;
#5409=ADVANCED_FACE('',(#684),#444,.T.) ;
#5410=ADVANCED_FACE('',(#685),#5171,.T.) ;
#5411=ADVANCED_FACE('',(#686),#5172,.F.) ;
#5412=ADVANCED_FACE('',(#687),#445,.T.) ;
#5413=ADVANCED_FACE('',(#688),#5173,.T.) ;
#5414=ADVANCED_FACE('',(#689),#446,.T.) ;
#5415=ADVANCED_FACE('',(#690),#5174,.F.) ;
#5416=ADVANCED_FACE('',(#691),#5175,.T.) ;
#5417=ADVANCED_FACE('',(#692),#447,.T.) ;
#5418=ADVANCED_FACE('',(#693),#5176,.F.) ;
#5419=ADVANCED_FACE('',(#694,#359,#360),#448,.T.) ;
#5420=ADVANCED_FACE('',(#695),#216,.T.) ;
#5421=ADVANCED_FACE('',(#696),#5177,.T.) ;
#5422=ADVANCED_FACE('',(#697),#217,.T.) ;
#5423=ADVANCED_FACE('',(#698),#5178,.T.) ;
#5424=ADVANCED_FACE('',(#699),#218,.T.) ;
#5425=ADVANCED_FACE('',(#700),#5179,.T.) ;
#5426=ADVANCED_FACE('',(#701),#219,.T.) ;
#5427=ADVANCED_FACE('',(#702),#5180,.T.) ;
#5428=ADVANCED_FACE('',(#703),#220,.T.) ;
#5429=ADVANCED_FACE('',(#704),#221,.T.) ;
#5430=ADVANCED_FACE('',(#705),#5181,.T.) ;
#5431=ADVANCED_FACE('',(#706),#222,.T.) ;
#5432=ADVANCED_FACE('',(#707),#5182,.T.) ;
#5433=ADVANCED_FACE('',(#708),#5183,.T.) ;
#5434=ADVANCED_FACE('',(#709),#223,.T.) ;
#5435=ADVANCED_FACE('',(#710),#224,.T.) ;
#5436=ADVANCED_FACE('',(#711),#5184,.T.) ;
#5437=ADVANCED_FACE('',(#712),#225,.T.) ;
#5438=ADVANCED_FACE('',(#713),#5185,.T.) ;
#5439=ADVANCED_FACE('',(#714),#5186,.T.) ;
#5440=ADVANCED_FACE('',(#715),#226,.T.) ;
#5441=ADVANCED_FACE('',(#716),#5187,.T.) ;
#5442=ADVANCED_FACE('',(#717),#227,.T.) ;
#5443=ADVANCED_FACE('',(#718),#228,.T.) ;
#5444=ADVANCED_FACE('',(#719),#5188,.T.) ;
#5445=ADVANCED_FACE('',(#720),#229,.T.) ;
#5446=ADVANCED_FACE('',(#721),#5189,.T.) ;
#5447=ADVANCED_FACE('',(#722),#107,.F.) ;
#5448=ADVANCED_FACE('',(#723),#5190,.T.) ;
#5449=ADVANCED_FACE('',(#724),#449,.T.) ;
#5450=ADVANCED_FACE('',(#725),#5191,.F.) ;
#5451=ADVANCED_FACE('',(#726),#450,.T.) ;
#5452=ADVANCED_FACE('',(#727),#5192,.F.) ;
#5453=ADVANCED_FACE('',(#728),#451,.T.) ;
#5454=ADVANCED_FACE('',(#729),#5193,.T.) ;
#5455=ADVANCED_FACE('',(#730),#452,.T.) ;
#5456=ADVANCED_FACE('',(#731),#5194,.F.) ;
#5457=ADVANCED_FACE('',(#732),#453,.T.) ;
#5458=ADVANCED_FACE('',(#733),#5195,.T.) ;
#5459=ADVANCED_FACE('',(#734),#454,.T.) ;
#5460=ADVANCED_FACE('',(#735),#455,.T.) ;
#5461=ADVANCED_FACE('',(#736),#5196,.T.) ;
#5462=ADVANCED_FACE('',(#737),#456,.T.) ;
#5463=ADVANCED_FACE('',(#738,#361,#362),#457,.F.) ;
#5464=ADVANCED_FACE('',(#739),#5197,.T.) ;
#5465=ADVANCED_FACE('',(#740),#230,.T.) ;
#5466=ADVANCED_FACE('',(#741),#5198,.T.) ;
#5467=ADVANCED_FACE('',(#742),#231,.T.) ;
#5468=ADVANCED_FACE('',(#743),#5199,.F.) ;
#5469=ADVANCED_FACE('',(#744),#458,.T.) ;
#5470=ADVANCED_FACE('',(#745),#232,.T.) ;
#5471=ADVANCED_FACE('',(#746),#233,.T.) ;
#5472=ADVANCED_FACE('',(#747),#5200,.T.) ;
#5473=ADVANCED_FACE('',(#748),#5201,.T.) ;
#5474=ADVANCED_FACE('',(#749),#5202,.F.) ;
#5475=ADVANCED_FACE('',(#750),#459,.T.) ;
#5476=ADVANCED_FACE('',(#751),#5203,.F.) ;
#5571=CLOSED_SHELL('',(#5375,#5376,#5377,#5378,#5379,#5380,#5381,#5382,
#5383,#5384,#5385,#5386,#5387,#5388,#5389,#5390,#5391,#5392,#5393,#5394,
#5395,#5396,#5397,#5398,#5399,#5400,#5401,#5402,#5403,#5404,#5405,#5406,
#5407,#5408,#5409,#5410,#5411,#5412,#5413,#5414,#5415,#5416,#5417,#5418,
#5419,#5420,#5421,#5422,#5423,#5424,#5425,#5426,#5427,#5428,#5429,#5430,
#5431,#5432,#5433,#5434,#5435,#5436,#5437,#5438,#5439,#5440,#5441,#5442,
#5443,#5444,#5445,#5446,#5447,#5448,#5449,#5450,#5451,#5452,#5453,#5454,
#5455,#5456,#5457,#5458,#5459,#5460,#5461,#5462,#5463,#5464,#5465,#5466,
#5467,#5468,#5469,#5470,#5471,#5472,#5473,#5474,#5475,#5476)) ;
#6038=AXIS2_PLACEMENT_3D('',#9450,#7167,#7168) ;
#6039=AXIS2_PLACEMENT_3D('',#9451,#7169,#7170) ;
#6040=AXIS2_PLACEMENT_3D('',#9492,#7173,#7174) ;
#6041=AXIS2_PLACEMENT_3D('',#9506,#7175,#7176) ;
#6042=AXIS2_PLACEMENT_3D('',#9507,#7177,#7178) ;
#6043=AXIS2_PLACEMENT_3D('',#9524,#7181,#7182) ;
#6044=AXIS2_PLACEMENT_3D('',#9526,#7183,#7184) ;
#6045=AXIS2_PLACEMENT_3D('',#9540,#7185,#7186) ;
#6046=AXIS2_PLACEMENT_3D('',#9541,#7187,#7188) ;
#6047=AXIS2_PLACEMENT_3D('',#9558,#7191,#7192) ;
#6048=AXIS2_PLACEMENT_3D('',#9587,#7193,#7194) ;
#6049=AXIS2_PLACEMENT_3D('',#9601,#7195,#7196) ;
#6050=AXIS2_PLACEMENT_3D('',#9602,#7197,#7198) ;
#6051=AXIS2_PLACEMENT_3D('',#9619,#7201,#7202) ;
#6052=AXIS2_PLACEMENT_3D('',#9621,#7203,#7204) ;
#6053=AXIS2_PLACEMENT_3D('',#9635,#7205,#7206) ;
#6054=AXIS2_PLACEMENT_3D('',#9636,#7207,#7208) ;
#6055=AXIS2_PLACEMENT_3D('',#9666,#7211,#7212) ;
#6056=AXIS2_PLACEMENT_3D('',#9668,#7213,#7214) ;
#6057=AXIS2_PLACEMENT_3D('',#9682,#7215,#7216) ;
#6058=AXIS2_PLACEMENT_3D('',#9683,#7217,#7218) ;
#6059=AXIS2_PLACEMENT_3D('',#9731,#7221,#7222) ;
#6060=AXIS2_PLACEMENT_3D('',#9763,#7225,#7226) ;
#6061=AXIS2_PLACEMENT_3D('',#9764,#7227,#7228) ;
#6062=AXIS2_PLACEMENT_3D('',#9766,#7229,#7230) ;
#6063=AXIS2_PLACEMENT_3D('',#9780,#7231,#7232) ;
#6064=AXIS2_PLACEMENT_3D('',#9781,#7233,#7234) ;
#6065=AXIS2_PLACEMENT_3D('',#9783,#7235,#7236) ;
#6066=AXIS2_PLACEMENT_3D('',#9810,#7237,#7238) ;
#6067=AXIS2_PLACEMENT_3D('',#9811,#7239,#7240) ;
#6068=AXIS2_PLACEMENT_3D('',#9813,#7241,#7242) ;
#6069=AXIS2_PLACEMENT_3D('',#9827,#7243,#7244) ;
#6070=AXIS2_PLACEMENT_3D('',#9828,#7245,#7246) ;
#6071=AXIS2_PLACEMENT_3D('',#9857,#7247,#7248) ;
#6072=AXIS2_PLACEMENT_3D('',#9859,#7249,#7250) ;
#6073=AXIS2_PLACEMENT_3D('',#9860,#7251,#7252) ;
#6074=AXIS2_PLACEMENT_3D('',#9861,#7253,#7254) ;
#6075=AXIS2_PLACEMENT_3D('',#9864,#7257,#7258) ;
#6076=AXIS2_PLACEMENT_3D('',#9867,#7261,#7262) ;
#6077=AXIS2_PLACEMENT_3D('',#9884,#7265,#7266) ;
#6078=AXIS2_PLACEMENT_3D('',#9912,#7267,#7268) ;
#6079=AXIS2_PLACEMENT_3D('',#9913,#7269,#7270) ;
#6080=AXIS2_PLACEMENT_3D('',#9914,#7271,#7272) ;
#6081=AXIS2_PLACEMENT_3D('',#9916,#7273,#7274) ;
#6082=AXIS2_PLACEMENT_3D('',#9918,#7275,#7276) ;
#6083=AXIS2_PLACEMENT_3D('',#9933,#7277,#7278) ;
#6084=AXIS2_PLACEMENT_3D('',#9936,#7281,#7282) ;
#6085=AXIS2_PLACEMENT_3D('',#9938,#7283,#7284) ;
#6086=AXIS2_PLACEMENT_3D('',#9940,#7285,#7286) ;
#6087=AXIS2_PLACEMENT_3D('',#9941,#7287,#7288) ;
#6088=AXIS2_PLACEMENT_3D('',#9942,#7289,#7290) ;
#6089=AXIS2_PLACEMENT_3D('',#9945,#7293,#7294) ;
#6090=AXIS2_PLACEMENT_3D('',#9947,#7295,#7296) ;
#6091=AXIS2_PLACEMENT_3D('',#9949,#7297,#7298) ;
#6092=AXIS2_PLACEMENT_3D('',#9964,#7299,#7300) ;
#6093=AXIS2_PLACEMENT_3D('',#9983,#7303,#7304) ;
#6094=AXIS2_PLACEMENT_3D('',#9985,#7305,#7306) ;
#6095=AXIS2_PLACEMENT_3D('',#10001,#7307,#7308) ;
#6096=AXIS2_PLACEMENT_3D('',#10002,#7309,#7310) ;
#6097=AXIS2_PLACEMENT_3D('',#10019,#7313,#7314) ;
#6098=AXIS2_PLACEMENT_3D('',#10020,#7315,#7316) ;
#6099=AXIS2_PLACEMENT_3D('',#10021,#7317,#7318) ;
#6100=AXIS2_PLACEMENT_3D('',#10022,#7319,#7320) ;
#6101=AXIS2_PLACEMENT_3D('',#10026,#7322,#7323) ;
#6102=AXIS2_PLACEMENT_3D('',#10028,#7325,#7326) ;
#6103=AXIS2_PLACEMENT_3D('',#10032,#7329,#7330) ;
#6104=AXIS2_PLACEMENT_3D('',#10035,#7332,#7333) ;
#6105=AXIS2_PLACEMENT_3D('',#10036,#7334,#7335) ;
#6106=AXIS2_PLACEMENT_3D('',#10040,#7338,#7339) ;
#6107=AXIS2_PLACEMENT_3D('',#10043,#7341,#7342) ;
#6108=AXIS2_PLACEMENT_3D('',#10044,#7343,#7344) ;
#6109=AXIS2_PLACEMENT_3D('',#10048,#7347,#7348) ;
#6110=AXIS2_PLACEMENT_3D('',#10051,#7350,#7351) ;
#6111=AXIS2_PLACEMENT_3D('',#10052,#7352,#7353) ;
#6112=AXIS2_PLACEMENT_3D('',#10055,#7355,#7356) ;
#6113=AXIS2_PLACEMENT_3D('',#10056,#7357,#7358) ;
#6114=AXIS2_PLACEMENT_3D('',#10060,#7361,#7362) ;
#6115=AXIS2_PLACEMENT_3D('',#10063,#7364,#7365) ;
#6116=AXIS2_PLACEMENT_3D('',#10064,#7366,#7367) ;
#6117=AXIS2_PLACEMENT_3D('',#10068,#7370,#7371) ;
#6118=AXIS2_PLACEMENT_3D('',#10071,#7373,#7374) ;
#6119=AXIS2_PLACEMENT_3D('',#10072,#7375,#7376) ;
#6120=AXIS2_PLACEMENT_3D('',#10075,#7378,#7379) ;
#6121=AXIS2_PLACEMENT_3D('',#10076,#7380,#7381) ;
#6122=AXIS2_PLACEMENT_3D('',#10080,#7384,#7385) ;
#6123=AXIS2_PLACEMENT_3D('',#10083,#7387,#7388) ;
#6124=AXIS2_PLACEMENT_3D('',#10084,#7389,#7390) ;
#6125=AXIS2_PLACEMENT_3D('',#10089,#7392,#7393) ;
#6126=AXIS2_PLACEMENT_3D('',#10092,#7395,#7396) ;
#6127=AXIS2_PLACEMENT_3D('',#10094,#7397,#7398) ;
#6128=AXIS2_PLACEMENT_3D('',#10095,#7399,#7400) ;
#6129=AXIS2_PLACEMENT_3D('',#10098,#7401,#7402) ;
#6130=AXIS2_PLACEMENT_3D('',#10123,#7403,#7404) ;
#6131=AXIS2_PLACEMENT_3D('',#10142,#7407,#7408) ;
#6132=AXIS2_PLACEMENT_3D('',#10144,#7409,#7410) ;
#6133=AXIS2_PLACEMENT_3D('',#10158,#7411,#7412) ;
#6134=AXIS2_PLACEMENT_3D('',#10159,#7413,#7414) ;
#6135=AXIS2_PLACEMENT_3D('',#10176,#7417,#7418) ;
#6136=AXIS2_PLACEMENT_3D('',#10178,#7419,#7420) ;
#6137=AXIS2_PLACEMENT_3D('',#10192,#7421,#7422) ;
#6138=AXIS2_PLACEMENT_3D('',#10193,#7423,#7424) ;
#6139=AXIS2_PLACEMENT_3D('',#10234,#7426,#7427) ;
#6140=AXIS2_PLACEMENT_3D('',#10263,#7428,#7429) ;
#6141=AXIS2_PLACEMENT_3D('',#10265,#7430,#7431) ;
#6142=AXIS2_PLACEMENT_3D('',#10266,#7432,#7433) ;
#6143=AXIS2_PLACEMENT_3D('',#10267,#7434,#7435) ;
#6144=AXIS2_PLACEMENT_3D('',#10286,#7438,#7439) ;
#6145=AXIS2_PLACEMENT_3D('',#10313,#7440,#7441) ;
#6146=AXIS2_PLACEMENT_3D('',#10314,#7442,#7443) ;
#6147=AXIS2_PLACEMENT_3D('',#10316,#7444,#7445) ;
#6148=AXIS2_PLACEMENT_3D('',#10330,#7446,#7447) ;
#6149=AXIS2_PLACEMENT_3D('',#10331,#7448,#7449) ;
#6150=AXIS2_PLACEMENT_3D('',#10335,#7451,#7452) ;
#6151=AXIS2_PLACEMENT_3D('',#10337,#7454,#7455) ;
#6152=AXIS2_PLACEMENT_3D('',#10365,#7456,#7457) ;
#6153=AXIS2_PLACEMENT_3D('',#10366,#7458,#7459) ;
#6154=AXIS2_PLACEMENT_3D('',#10367,#7460,#7461) ;
#6155=AXIS2_PLACEMENT_3D('',#10397,#7464,#7465) ;
#6156=AXIS2_PLACEMENT_3D('',#10412,#7467,#7468) ;
#6157=AXIS2_PLACEMENT_3D('',#10440,#7469,#7470) ;
#6158=AXIS2_PLACEMENT_3D('',#10441,#7471,#7472) ;
#6159=AXIS2_PLACEMENT_3D('',#10442,#7473,#7474) ;
#6160=AXIS2_PLACEMENT_3D('',#10444,#7475,#7476) ;
#6161=AXIS2_PLACEMENT_3D('',#10457,#7477,#7478) ;
#6162=AXIS2_PLACEMENT_3D('',#10460,#7481,#7482) ;
#6163=AXIS2_PLACEMENT_3D('',#10462,#7483,#7484) ;
#6164=AXIS2_PLACEMENT_3D('',#10475,#7485,#7486) ;
#6165=AXIS2_PLACEMENT_3D('',#10477,#7488,#7489) ;
#6166=AXIS2_PLACEMENT_3D('',#10507,#7492,#7493) ;
#6167=AXIS2_PLACEMENT_3D('',#10509,#7494,#7495) ;
#6168=AXIS2_PLACEMENT_3D('',#10522,#7496,#7497) ;
#6169=AXIS2_PLACEMENT_3D('',#10539,#7500,#7501) ;
#6170=AXIS2_PLACEMENT_3D('',#10540,#7502,#7503) ;
#6171=AXIS2_PLACEMENT_3D('',#10541,#7504,#7505) ;
#6172=AXIS2_PLACEMENT_3D('',#10542,#7506,#7507) ;
#6173=AXIS2_PLACEMENT_3D('',#10544,#7508,#7509) ;
#6174=AXIS2_PLACEMENT_3D('',#10557,#7510,#7511) ;
#6175=AXIS2_PLACEMENT_3D('',#10572,#7513,#7514) ;
#6176=AXIS2_PLACEMENT_3D('',#10574,#7515,#7516) ;
#6177=AXIS2_PLACEMENT_3D('',#10587,#7517,#7518) ;
#6178=AXIS2_PLACEMENT_3D('',#10612,#7520,#7521) ;
#6179=AXIS2_PLACEMENT_3D('',#10625,#7522,#7523) ;
#6180=AXIS2_PLACEMENT_3D('',#10627,#7525,#7526) ;
#6181=AXIS2_PLACEMENT_3D('',#10629,#7528,#7529) ;
#6182=AXIS2_PLACEMENT_3D('',#10631,#7531,#7532) ;
#6183=AXIS2_PLACEMENT_3D('',#10633,#7534,#7535) ;
#6184=AXIS2_PLACEMENT_3D('',#10635,#7537,#7538) ;
#6185=AXIS2_PLACEMENT_3D('',#10637,#7540,#7541) ;
#6186=AXIS2_PLACEMENT_3D('',#10639,#7543,#7544) ;
#6187=AXIS2_PLACEMENT_3D('',#10641,#7546,#7547) ;
#6188=AXIS2_PLACEMENT_3D('',#10643,#7549,#7550) ;
#6189=AXIS2_PLACEMENT_3D('',#10645,#7552,#7553) ;
#6190=AXIS2_PLACEMENT_3D('',#10647,#7555,#7556) ;
#6191=AXIS2_PLACEMENT_3D('',#10649,#7558,#7559) ;
#6192=AXIS2_PLACEMENT_3D('',#10651,#7561,#7562) ;
#6193=AXIS2_PLACEMENT_3D('',#10653,#7564,#7565) ;
#6194=AXIS2_PLACEMENT_3D('',#10654,#7566,#7567) ;
#6195=AXIS2_PLACEMENT_3D('',#10657,#7568,#7569) ;
#6196=AXIS2_PLACEMENT_3D('',#10661,#7571,#7572) ;
#6197=AXIS2_PLACEMENT_3D('',#10664,#7574,#7575) ;
#6198=AXIS2_PLACEMENT_3D('',#10665,#7576,#7577) ;
#6199=AXIS2_PLACEMENT_3D('',#10693,#7579,#7580) ;
#6200=AXIS2_PLACEMENT_3D('',#10707,#7581,#7582) ;
#6201=AXIS2_PLACEMENT_3D('',#10708,#7583,#7584) ;
#6202=AXIS2_PLACEMENT_3D('',#10723,#7586,#7587) ;
#6203=AXIS2_PLACEMENT_3D('',#10724,#7588,#7589) ;
#6204=AXIS2_PLACEMENT_3D('',#10725,#7590,#7591) ;
#6205=AXIS2_PLACEMENT_3D('',#10729,#7593,#7594) ;
#6206=AXIS2_PLACEMENT_3D('',#10731,#7596,#7597) ;
#6207=AXIS2_PLACEMENT_3D('',#10735,#7600,#7601) ;
#6208=AXIS2_PLACEMENT_3D('',#10737,#7602,#7603) ;
#6209=AXIS2_PLACEMENT_3D('',#10762,#7604,#7605) ;
#6210=AXIS2_PLACEMENT_3D('',#10787,#7606,#7607) ;
#6211=AXIS2_PLACEMENT_3D('',#10789,#7609,#7610) ;
#6212=AXIS2_PLACEMENT_3D('',#10790,#7611,#7612) ;
#6213=AXIS2_PLACEMENT_3D('',#10792,#7614,#7615) ;
#6214=AXIS2_PLACEMENT_3D('',#10794,#7617,#7618) ;
#7167=DIRECTION('axis',(0.,0.,1.)) ;
#7168=DIRECTION('refdir',(1.,0.,0.)) ;
#7169=DIRECTION('center_axis',(0.,0.,-1.)) ;
#7170=DIRECTION('ref_axis',(0.707106781186546,-0.707106781186549,0.)) ;
#7171=DIRECTION('',(0.,0.,1.)) ;
#7172=DIRECTION('',(0.,0.,-1.)) ;
#7173=DIRECTION('center_axis',(-1.,0.,0.)) ;
#7174=DIRECTION('ref_axis',(0.,-0.813733471206731,0.581238193719102)) ;
#7175=DIRECTION('center_axis',(1.,0.,0.)) ;
#7176=DIRECTION('ref_axis',(0.,-0.813733471206731,0.581238193719102)) ;
#7177=DIRECTION('center_axis',(0.,-0.940315265291054,-0.340304572200573)) ;
#7178=DIRECTION('ref_axis',(0.707106781186547,-0.240631670671808,0.664903300540534)) ;
#7179=DIRECTION('',(0.,0.940315265291054,0.340304572200573)) ;
#7180=DIRECTION('',(0.,-0.940315265291054,-0.340304572200573)) ;
#7181=DIRECTION('center_axis',(-1.,0.,0.)) ;
#7182=DIRECTION('ref_axis',(0.,0.,1.)) ;
#7183=DIRECTION('center_axis',(1.,0.,0.)) ;
#7184=DIRECTION('ref_axis',(0.,0.554700196225229,-0.832050294337844)) ;
#7185=DIRECTION('center_axis',(-1.,0.,0.)) ;
#7186=DIRECTION('ref_axis',(0.,0.554700196225229,-0.832050294337844)) ;
#7187=DIRECTION('center_axis',(0.,-0.561501418337265,-0.827475774391758)) ;
#7188=DIRECTION('ref_axis',(0.707106781186551,-0.585113731339998,0.397041460552144)) ;
#7189=DIRECTION('',(0.,0.561501418337265,0.827475774391758)) ;
#7190=DIRECTION('',(0.,-0.561501418337265,-0.827475774391758)) ;
#7191=DIRECTION('center_axis',(1.,0.,0.)) ;
#7192=DIRECTION('ref_axis',(0.,0.,-1.)) ;
#7193=DIRECTION('center_axis',(-1.,0.,0.)) ;
#7194=DIRECTION('ref_axis',(0.,-0.86974260015344,-0.493505632671334)) ;
#7195=DIRECTION('center_axis',(1.,0.,0.)) ;
#7196=DIRECTION('ref_axis',(0.,-0.86974260015344,-0.493505632671334)) ;
#7197=DIRECTION('center_axis',(0.,0.239567708183828,-0.970879659481827)) ;
#7198=DIRECTION('ref_axis',(0.707106781186544,-0.68651559093569,-0.169399951010105)) ;
#7199=DIRECTION('',(0.,0.239567708183828,-0.970879659481827)) ;
#7200=DIRECTION('',(0.,-0.239567708183828,0.970879659481827)) ;
#7201=DIRECTION('center_axis',(1.,0.,0.)) ;
#7202=DIRECTION('ref_axis',(0.,0.,-1.)) ;
#7203=DIRECTION('center_axis',(-1.,0.,0.)) ;
#7204=DIRECTION('ref_axis',(0.,-0.570395809495344,0.821369965673296)) ;
#7205=DIRECTION('center_axis',(1.,0.,0.)) ;
#7206=DIRECTION('ref_axis',(0.,-0.570395809495344,0.821369965673296)) ;
#7207=DIRECTION('center_axis',(0.,0.707106781186548,-0.707106781186548)) ;
#7208=DIRECTION('ref_axis',(0.707106781186552,-0.499999999999989,-0.500000000000005)) ;
#7209=DIRECTION('',(0.,0.707106781186548,-0.707106781186548)) ;
#7210=DIRECTION('',(0.,-0.707106781186548,0.707106781186548)) ;
#7211=DIRECTION('center_axis',(-1.,0.,0.)) ;
#7212=DIRECTION('ref_axis',(0.,0.707106781186552,-0.707106781186543)) ;
#7213=DIRECTION('center_axis',(1.,0.,0.)) ;
#7214=DIRECTION('ref_axis',(0.,0.707106781186551,-0.707106781186544)) ;
#7215=DIRECTION('center_axis',(-1.,0.,0.)) ;
#7216=DIRECTION('ref_axis',(0.,0.707106781186551,-0.707106781186544)) ;
#7217=DIRECTION('center_axis',(0.,0.,1.)) ;
#7218=DIRECTION('ref_axis',(0.707106781186548,0.707106781186548,0.)) ;
#7219=DIRECTION('',(0.,0.,-1.)) ;
#7220=DIRECTION('',(0.,0.,1.)) ;
#7221=DIRECTION('center_axis',(0.,0.0518000861243686,0.998657474351195)) ;
#7222=DIRECTION('ref_axis',(0.707106781186548,0.70615747219636,-0.0366281921646092)) ;
#7223=DIRECTION('',(0.,0.0518000861243686,0.998657474351195)) ;
#7224=DIRECTION('',(0.,-0.0518000861243686,-0.998657474351195)) ;
#7225=DIRECTION('center_axis',(0.,0.060701587016572,0.998155958422164)) ;
#7226=DIRECTION('ref_axis',(0.,0.998155958422164,-0.060701587016572)) ;
#7227=DIRECTION('center_axis',(-1.,0.,0.)) ;
#7228=DIRECTION('ref_axis',(0.,0.,1.)) ;
#7229=DIRECTION('center_axis',(1.,0.,0.)) ;
#7230=DIRECTION('ref_axis',(0.,-0.860291533634174,-0.509802390301733)) ;
#7231=DIRECTION('center_axis',(-1.,0.,0.)) ;
#7232=DIRECTION('ref_axis',(0.,-0.860291533634174,-0.509802390301733)) ;
#7233=DIRECTION('center_axis',(1.,0.,0.)) ;
#7234=DIRECTION('ref_axis',(0.,0.,-1.)) ;
#7235=DIRECTION('center_axis',(1.,0.,0.)) ;
#7236=DIRECTION('ref_axis',(0.,0.933269707299496,0.359176354228828)) ;
#7237=DIRECTION('center_axis',(-1.,0.,0.)) ;
#7238=DIRECTION('ref_axis',(0.,0.933269707299496,0.359176354228828)) ;
#7239=DIRECTION('center_axis',(1.,0.,0.)) ;
#7240=DIRECTION('ref_axis',(0.,0.,-1.)) ;
#7241=DIRECTION('center_axis',(-1.,0.,0.)) ;
#7242=DIRECTION('ref_axis',(0.,0.867757267880784,0.49698825342263)) ;
#7243=DIRECTION('center_axis',(1.,0.,0.)) ;
#7244=DIRECTION('ref_axis',(0.,0.867757267880784,0.49698825342263)) ;
#7245=DIRECTION('center_axis',(-1.,0.,0.)) ;
#7246=DIRECTION('ref_axis',(0.,0.,1.)) ;
#7247=DIRECTION('center_axis',(1.,0.,0.)) ;
#7248=DIRECTION('ref_axis',(0.,-0.923683059121558,-0.383157417117091)) ;
#7249=DIRECTION('center_axis',(0.,-0.706713794874047,0.707499549211675)) ;
#7250=DIRECTION('ref_axis',(1.,0.,0.)) ;
#7251=DIRECTION('center_axis',(-1.,0.,0.)) ;
#7252=DIRECTION('ref_axis',(0.,-0.923683059121558,-0.383157417117091)) ;
#7253=DIRECTION('center_axis',(0.,0.,1.)) ;
#7254=DIRECTION('ref_axis',(0.70710678118654,0.707106781186555,0.)) ;
#7255=DIRECTION('',(0.,0.,-1.)) ;
#7256=DIRECTION('',(0.,0.,1.)) ;
#7257=DIRECTION('center_axis',(0.,-0.707106781186548,0.707106781186548)) ;
#7258=DIRECTION('ref_axis',(0.707106781186552,0.499999999999989,0.500000000000005)) ;
#7259=DIRECTION('',(0.,-0.707106781186548,0.707106781186548)) ;
#7260=DIRECTION('',(0.,0.707106781186548,-0.707106781186548)) ;
#7261=DIRECTION('center_axis',(0.,0.0695982628490372,0.997575100836221)) ;
#7262=DIRECTION('ref_axis',(0.707106781186555,0.705392118544138,-0.049213403619365)) ;
#7263=DIRECTION('',(0.,0.0695982628490372,0.997575100836221)) ;
#7264=DIRECTION('',(0.,-0.0695982628490372,-0.997575100836221)) ;
#7265=DIRECTION('center_axis',(1.,0.,0.)) ;
#7266=DIRECTION('ref_axis',(0.,4.0179797404504E-5,0.999999999192792)) ;
#7267=DIRECTION('center_axis',(-1.,0.,0.)) ;
#7268=DIRECTION('ref_axis',(0.,0.,1.)) ;
#7269=DIRECTION('center_axis',(1.,0.,0.)) ;
#7270=DIRECTION('ref_axis',(0.,0.,1.)) ;
#7271=DIRECTION('center_axis',(1.,0.,0.)) ;
#7272=DIRECTION('ref_axis',(0.,0.,-1.)) ;
#7273=DIRECTION('center_axis',(1.,0.,0.)) ;
#7274=DIRECTION('ref_axis',(0.,-0.649652327582147,-0.760231447170596)) ;
#7275=DIRECTION('center_axis',(-1.,0.,0.)) ;
#7276=DIRECTION('ref_axis',(0.,-0.649652327582147,-0.760231447170596)) ;
#7277=DIRECTION('center_axis',(0.,0.,-1.)) ;
#7278=DIRECTION('ref_axis',(0.707106781186548,-0.707106781186548,0.)) ;
#7279=DIRECTION('',(0.,0.,1.)) ;
#7280=DIRECTION('',(0.,0.,-1.)) ;
#7281=DIRECTION('center_axis',(-1.,0.,0.)) ;
#7282=DIRECTION('ref_axis',(0.,0.,1.)) ;
#7283=DIRECTION('center_axis',(-1.,0.,0.)) ;
#7284=DIRECTION('ref_axis',(0.,0.929577903322658,0.368625720283123)) ;
#7285=DIRECTION('center_axis',(0.,0.0262932027111255,0.999654273982356)) ;
#7286=DIRECTION('ref_axis',(0.,-0.999654273982356,0.0262932027111255)) ;
#7287=DIRECTION('center_axis',(1.,0.,0.)) ;
#7288=DIRECTION('ref_axis',(0.,0.929577903322658,0.368625720283123)) ;
#7289=DIRECTION('center_axis',(0.,-0.0257899447975391,-0.999667384056987)) ;
#7290=DIRECTION('ref_axis',(0.707106781186539,-0.706871586197721,0.0182362448527659)) ;
#7291=DIRECTION('',(0.,0.0257899447975391,0.999667384056987)) ;
#7292=DIRECTION('',(0.,-0.0257899447975391,-0.999667384056987)) ;
#7293=DIRECTION('center_axis',(-1.,0.,0.)) ;
#7294=DIRECTION('ref_axis',(0.,0.,1.)) ;
#7295=DIRECTION('center_axis',(-1.,0.,0.)) ;
#7296=DIRECTION('ref_axis',(0.,0.906183139995266,0.422885465331122)) ;
#7297=DIRECTION('center_axis',(1.,0.,0.)) ;
#7298=DIRECTION('ref_axis',(0.,0.906183139995266,0.422885465331122)) ;
#7299=DIRECTION('center_axis',(0.,0.863187603129405,-0.504883315037953)) ;
#7300=DIRECTION('ref_axis',(0.707106781186553,-0.357006415771267,-0.610365807608966)) ;
#7301=DIRECTION('',(0.,0.863187603129405,-0.504883315037953)) ;
#7302=DIRECTION('',(0.,-0.863187603129405,0.504883315037953)) ;
#7303=DIRECTION('center_axis',(-1.,0.,0.)) ;
#7304=DIRECTION('ref_axis',(0.,0.,1.)) ;
#7305=DIRECTION('center_axis',(1.,0.,0.)) ;
#7306=DIRECTION('ref_axis',(0.,-0.0970999642854239,0.995274633925616)) ;
#7307=DIRECTION('center_axis',(-1.,0.,0.)) ;
#7308=DIRECTION('ref_axis',(0.,-0.0970999642854239,0.995274633925616)) ;
#7309=DIRECTION('center_axis',(0.,0.940190624657783,0.340648777049922)) ;
#7310=DIRECTION('ref_axis',(0.70710678118655,0.240875060254906,-0.664815166303532)) ;
#7311=DIRECTION('',(0.,0.940190624657783,0.340648777049922)) ;
#7312=DIRECTION('',(0.,-0.940190624657783,-0.340648777049922)) ;
#7313=DIRECTION('center_axis',(1.,0.,0.)) ;
#7314=DIRECTION('ref_axis',(0.,0.,-1.)) ;
#7315=DIRECTION('center_axis',(1.,0.,0.)) ;
#7316=DIRECTION('ref_axis',(0.,-0.624695047554424,-0.780868809443031)) ;
#7317=DIRECTION('center_axis',(-1.,0.,0.)) ;
#7318=DIRECTION('ref_axis',(0.,-0.624695047554424,-0.780868809443031)) ;
#7319=DIRECTION('center_axis',(1.,0.,0.)) ;
#7320=DIRECTION('ref_axis',(0.,-0.987974784374397,-0.154615088010078)) ;
#7321=DIRECTION('',(1.,0.,0.)) ;
#7322=DIRECTION('center_axis',(-1.,0.,0.)) ;
#7323=DIRECTION('ref_axis',(0.,-0.624695047554424,-0.780868809443031)) ;
#7324=DIRECTION('',(1.,0.,0.)) ;
#7325=DIRECTION('center_axis',(0.,-1.,0.)) ;
#7326=DIRECTION('ref_axis',(0.,0.,-1.)) ;
#7327=DIRECTION('',(1.,0.,0.)) ;
#7328=DIRECTION('',(0.,0.,1.)) ;
#7329=DIRECTION('center_axis',(1.,0.,0.)) ;
#7330=DIRECTION('ref_axis',(0.,-0.244681224382906,0.969603577981477)) ;
#7331=DIRECTION('',(1.,0.,0.)) ;
#7332=DIRECTION('center_axis',(-1.,0.,0.)) ;
#7333=DIRECTION('ref_axis',(0.,-0.813733471206731,0.581238193719102)) ;
#7334=DIRECTION('center_axis',(0.,-0.340304572200573,0.940315265291054)) ;
#7335=DIRECTION('ref_axis',(0.,-0.940315265291054,-0.340304572200573)) ;
#7336=DIRECTION('',(1.,0.,0.)) ;
#7337=DIRECTION('',(0.,0.940315265291054,0.340304572200573)) ;
#7338=DIRECTION('center_axis',(1.,0.,0.)) ;
#7339=DIRECTION('ref_axis',(0.,0.361292570457734,-0.932452507386861)) ;
#7340=DIRECTION('',(1.,0.,0.)) ;
#7341=DIRECTION('center_axis',(1.,0.,0.)) ;
#7342=DIRECTION('ref_axis',(0.,0.554700196225229,-0.832050294337844)) ;
#7343=DIRECTION('center_axis',(0.,-0.827475774391758,0.561501418337265)) ;
#7344=DIRECTION('ref_axis',(0.,-0.561501418337265,-0.827475774391758)) ;
#7345=DIRECTION('',(1.,0.,0.)) ;
#7346=DIRECTION('',(0.,0.561501418337265,0.827475774391758)) ;
#7347=DIRECTION('center_axis',(1.,0.,0.)) ;
#7348=DIRECTION('ref_axis',(0.,-0.0509372265161325,0.998701856889655)) ;
#7349=DIRECTION('',(1.,0.,0.)) ;
#7350=DIRECTION('center_axis',(-1.,0.,0.)) ;
#7351=DIRECTION('ref_axis',(0.,-0.570395809495344,0.821369965673296)) ;
#7352=DIRECTION('center_axis',(1.,0.,0.)) ;
#7353=DIRECTION('ref_axis',(0.,-0.0803728928848199,-0.996764865998659)) ;
#7354=DIRECTION('',(1.,0.,0.)) ;
#7355=DIRECTION('center_axis',(1.,0.,0.)) ;
#7356=DIRECTION('ref_axis',(0.,0.707106781186551,-0.707106781186544)) ;
#7357=DIRECTION('center_axis',(0.,-1.,0.)) ;
#7358=DIRECTION('ref_axis',(0.,0.,-1.)) ;
#7359=DIRECTION('',(1.,0.,0.)) ;
#7360=DIRECTION('',(0.,0.,1.)) ;
#7361=DIRECTION('center_axis',(1.,0.,0.)) ;
#7362=DIRECTION('ref_axis',(0.,0.999964987220335,0.0083680543398295)) ;
#7363=DIRECTION('',(1.,0.,0.)) ;
#7364=DIRECTION('center_axis',(-1.,0.,0.)) ;
#7365=DIRECTION('ref_axis',(0.,0.,1.)) ;
#7366=DIRECTION('center_axis',(0.,1.,0.)) ;
#7367=DIRECTION('ref_axis',(0.,0.,1.)) ;
#7368=DIRECTION('',(1.,0.,0.)) ;
#7369=DIRECTION('',(0.,0.,-1.)) ;
#7370=DIRECTION('center_axis',(1.,0.,0.)) ;
#7371=DIRECTION('ref_axis',(0.,-0.998538306838623,-0.0540485871772473)) ;
#7372=DIRECTION('',(1.,0.,0.)) ;
#7373=DIRECTION('center_axis',(1.,0.,0.)) ;
#7374=DIRECTION('ref_axis',(0.,-0.860291533634174,-0.509802390301733)) ;
#7375=DIRECTION('center_axis',(1.,0.,0.)) ;
#7376=DIRECTION('ref_axis',(0.,0.999980636834705,0.00622301821128131)) ;
#7377=DIRECTION('',(1.,0.,0.)) ;
#7378=DIRECTION('center_axis',(-1.,0.,0.)) ;
#7379=DIRECTION('ref_axis',(0.,0.867757267880784,0.49698825342263)) ;
#7380=DIRECTION('center_axis',(0.,1.,0.)) ;
#7381=DIRECTION('ref_axis',(0.,0.,1.)) ;
#7382=DIRECTION('',(1.,0.,0.)) ;
#7383=DIRECTION('',(0.,0.,-1.)) ;
#7384=DIRECTION('center_axis',(1.,0.,0.)) ;
#7385=DIRECTION('ref_axis',(0.,-0.999998748960749,-0.00158179547895617)) ;
#7386=DIRECTION('',(1.,0.,0.)) ;
#7387=DIRECTION('center_axis',(1.,0.,0.)) ;
#7388=DIRECTION('ref_axis',(0.,-0.923683059121558,-0.383157417117091)) ;
#7389=DIRECTION('center_axis',(1.,0.,0.)) ;
#7390=DIRECTION('ref_axis',(0.,0.,-1.)) ;
#7391=DIRECTION('',(0.,0.,1.)) ;
#7392=DIRECTION('center_axis',(1.,0.,0.)) ;
#7393=DIRECTION('ref_axis',(0.,0.,-1.)) ;
#7394=DIRECTION('',(0.,0.,-1.)) ;
#7395=DIRECTION('center_axis',(1.,0.,0.)) ;
#7396=DIRECTION('ref_axis',(0.,3.41514000732436E-15,1.)) ;
#7397=DIRECTION('center_axis',(-1.,0.,0.)) ;
#7398=DIRECTION('ref_axis',(0.,0.,-1.)) ;
#7399=DIRECTION('center_axis',(1.,0.,0.)) ;
#7400=DIRECTION('ref_axis',(0.,0.,-1.)) ;
#7401=DIRECTION('center_axis',(1.,0.,0.)) ;
#7402=DIRECTION('ref_axis',(0.,-0.624695047554424,-0.780868809443031)) ;
#7403=DIRECTION('center_axis',(0.,0.940190624657783,0.340648777049922)) ;
#7404=DIRECTION('ref_axis',(-0.707106781186527,0.240875060254903,-0.664815166303557)) ;
#7405=DIRECTION('',(0.,0.940190624657783,0.340648777049922)) ;
#7406=DIRECTION('',(0.,-0.940190624657783,-0.340648777049922)) ;
#7407=DIRECTION('center_axis',(1.,0.,0.)) ;
#7408=DIRECTION('ref_axis',(0.,-0.0927241376138027,0.995691837017748)) ;
#7409=DIRECTION('center_axis',(-1.,0.,0.)) ;
#7410=DIRECTION('ref_axis',(0.,-0.0970999642854239,0.995274633925616)) ;
#7411=DIRECTION('center_axis',(1.,0.,0.)) ;
#7412=DIRECTION('ref_axis',(0.,-0.0970999642854239,0.995274633925616)) ;
#7413=DIRECTION('center_axis',(0.,0.863187603129405,-0.504883315037953)) ;
#7414=DIRECTION('ref_axis',(-0.707106781186538,-0.357006415771298,-0.610365807608966)) ;
#7415=DIRECTION('',(0.,0.863187603129405,-0.504883315037953)) ;
#7416=DIRECTION('',(0.,-0.863187603129405,0.504883315037953)) ;
#7417=DIRECTION('center_axis',(1.,0.,0.)) ;
#7418=DIRECTION('ref_axis',(0.,0.,-1.)) ;
#7419=DIRECTION('center_axis',(-1.,0.,0.)) ;
#7420=DIRECTION('ref_axis',(0.,0.906183139995266,0.422885465331122)) ;
#7421=DIRECTION('center_axis',(1.,0.,0.)) ;
#7422=DIRECTION('ref_axis',(0.,0.906183139995266,0.422885465331122)) ;
#7423=DIRECTION('center_axis',(0.,0.,-1.)) ;
#7424=DIRECTION('ref_axis',(-0.707106781186532,-0.707106781186563,0.)) ;
#7425=DIRECTION('',(0.,0.,-1.)) ;
#7426=DIRECTION('center_axis',(1.,0.,0.)) ;
#7427=DIRECTION('ref_axis',(0.,0.,-1.)) ;
#7428=DIRECTION('center_axis',(-1.,0.,0.)) ;
#7429=DIRECTION('ref_axis',(0.,0.929577903322658,0.368625720283123)) ;
#7430=DIRECTION('center_axis',(0.,0.0262932027111255,0.999654273982356)) ;
#7431=DIRECTION('ref_axis',(-1.,0.,0.)) ;
#7432=DIRECTION('center_axis',(1.,0.,0.)) ;
#7433=DIRECTION('ref_axis',(0.,0.929577903322658,0.368625720283123)) ;
#7434=DIRECTION('center_axis',(0.,-0.0257899447975391,-0.999667384056987)) ;
#7435=DIRECTION('ref_axis',(-0.707106781186531,-0.706871586197729,0.0182362448527662)) ;
#7436=DIRECTION('',(0.,0.0257899447975391,0.999667384056987)) ;
#7437=DIRECTION('',(0.,-0.0257899447975391,-0.999667384056987)) ;
#7438=DIRECTION('center_axis',(1.,0.,0.)) ;
#7439=DIRECTION('ref_axis',(0.,-4.0179797404504E-5,0.999999999192792)) ;
#7440=DIRECTION('center_axis',(1.,0.,0.)) ;
#7441=DIRECTION('ref_axis',(0.,0.,1.)) ;
#7442=DIRECTION('center_axis',(1.,0.,0.)) ;
#7443=DIRECTION('ref_axis',(0.,0.,-1.)) ;
#7444=DIRECTION('center_axis',(1.,0.,0.)) ;
#7445=DIRECTION('ref_axis',(0.,-0.649652327582147,-0.760231447170596)) ;
#7446=DIRECTION('center_axis',(-1.,0.,0.)) ;
#7447=DIRECTION('ref_axis',(0.,-0.649652327582147,-0.760231447170596)) ;
#7448=DIRECTION('center_axis',(0.,0.0695982628490372,0.997575100836221)) ;
#7449=DIRECTION('ref_axis',(-0.707106781186547,0.705392118544146,-0.0492134036193656)) ;
#7450=DIRECTION('',(0.,0.0695982628490372,0.997575100836221)) ;
#7451=DIRECTION('center_axis',(0.,-0.060701587016572,-0.998155958422164)) ;
#7452=DIRECTION('ref_axis',(0.,-0.998155958422164,0.060701587016572)) ;
#7453=DIRECTION('',(0.,-0.0695982628490372,-0.997575100836221)) ;
#7454=DIRECTION('center_axis',(1.,0.,0.)) ;
#7455=DIRECTION('ref_axis',(0.,0.,-1.)) ;
#7456=DIRECTION('center_axis',(0.,-0.706713794874047,0.707499549211675)) ;
#7457=DIRECTION('ref_axis',(0.,0.707499549211675,0.706713794874047)) ;
#7458=DIRECTION('center_axis',(-1.,0.,0.)) ;
#7459=DIRECTION('ref_axis',(0.,-0.923683059121558,-0.383157417117091)) ;
#7460=DIRECTION('center_axis',(0.,-0.707106781186548,0.707106781186548)) ;
#7461=DIRECTION('ref_axis',(-0.707106781186544,0.499999999999995,0.50000000000001)) ;
#7462=DIRECTION('',(0.,-0.707106781186547,0.707106781186547)) ;
#7463=DIRECTION('',(0.,0.707106781186548,-0.707106781186548)) ;
#7464=DIRECTION('center_axis',(0.,0.,1.)) ;
#7465=DIRECTION('ref_axis',(-0.707106781186548,0.707106781186548,0.)) ;
#7466=DIRECTION('',(0.,0.,1.)) ;
#7467=DIRECTION('center_axis',(1.,0.,0.)) ;
#7468=DIRECTION('ref_axis',(0.,0.,-1.)) ;
#7469=DIRECTION('center_axis',(1.,0.,0.)) ;
#7470=DIRECTION('ref_axis',(0.,0.933269707299496,0.359176354228828)) ;
#7471=DIRECTION('center_axis',(-1.,0.,0.)) ;
#7472=DIRECTION('ref_axis',(0.,0.933269707299496,0.359176354228828)) ;
#7473=DIRECTION('center_axis',(1.,0.,0.)) ;
#7474=DIRECTION('ref_axis',(0.,0.,-1.)) ;
#7475=DIRECTION('center_axis',(1.,0.,0.)) ;
#7476=DIRECTION('ref_axis',(0.,0.867757267880784,0.49698825342263)) ;
#7477=DIRECTION('center_axis',(0.,0.0518000861243686,0.998657474351195)) ;
#7478=DIRECTION('ref_axis',(-0.70710678118654,0.706157472196368,-0.0366281921646096)) ;
#7479=DIRECTION('',(0.,0.0518000861243686,0.998657474351195)) ;
#7480=DIRECTION('',(0.,-0.0518000861243686,-0.998657474351195)) ;
#7481=DIRECTION('center_axis',(1.,0.,0.)) ;
#7482=DIRECTION('ref_axis',(0.,0.,-1.)) ;
#7483=DIRECTION('center_axis',(-1.,0.,0.)) ;
#7484=DIRECTION('ref_axis',(0.,-0.860291533634174,-0.509802390301733)) ;
#7485=DIRECTION('center_axis',(0.,0.,1.)) ;
#7486=DIRECTION('ref_axis',(-0.707106781186532,0.707106781186563,0.)) ;
#7487=DIRECTION('',(0.,0.,1.)) ;
#7488=DIRECTION('center_axis',(0.,0.707106781186548,-0.707106781186548)) ;
#7489=DIRECTION('ref_axis',(-0.707106781186544,-0.499999999999995,-0.50000000000001)) ;
#7490=DIRECTION('',(0.,0.707106781186548,-0.707106781186548)) ;
#7491=DIRECTION('',(0.,-0.707106781186548,0.707106781186548)) ;
#7492=DIRECTION('center_axis',(1.,0.,0.)) ;
#7493=DIRECTION('ref_axis',(0.,0.,-1.)) ;
#7494=DIRECTION('center_axis',(-1.,0.,0.)) ;
#7495=DIRECTION('ref_axis',(0.,0.707106781186551,-0.707106781186544)) ;
#7496=DIRECTION('center_axis',(0.,0.239567708183828,-0.970879659481827)) ;
#7497=DIRECTION('ref_axis',(-0.707106781186536,-0.686515590935697,-0.169399951010107)) ;
#7498=DIRECTION('',(0.,0.239567708183828,-0.970879659481827)) ;
#7499=DIRECTION('',(0.,-0.239567708183828,0.970879659481827)) ;
#7500=DIRECTION('center_axis',(1.,0.,0.)) ;
#7501=DIRECTION('ref_axis',(0.,0.,-1.)) ;
#7502=DIRECTION('center_axis',(-1.,0.,0.)) ;
#7503=DIRECTION('ref_axis',(0.,-0.86974260015344,-0.493505632671334)) ;
#7504=DIRECTION('center_axis',(1.,0.,0.)) ;
#7505=DIRECTION('ref_axis',(0.,-0.86974260015344,-0.493505632671334)) ;
#7506=DIRECTION('center_axis',(1.,0.,0.)) ;
#7507=DIRECTION('ref_axis',(0.,0.,-1.)) ;
#7508=DIRECTION('center_axis',(1.,0.,0.)) ;
#7509=DIRECTION('ref_axis',(0.,-0.570395809495344,0.821369965673296)) ;
#7510=DIRECTION('center_axis',(0.,-0.561501418337265,-0.827475774391758)) ;
#7511=DIRECTION('ref_axis',(-0.707106781186543,-0.585113731340005,0.397041460552148)) ;
#7512=DIRECTION('',(0.,-0.561501418337265,-0.827475774391758)) ;
#7513=DIRECTION('center_axis',(1.,0.,0.)) ;
#7514=DIRECTION('ref_axis',(0.,0.,-1.)) ;
#7515=DIRECTION('center_axis',(-1.,0.,0.)) ;
#7516=DIRECTION('ref_axis',(0.,0.554700196225229,-0.832050294337844)) ;
#7517=DIRECTION('center_axis',(0.,-0.940315265291054,-0.340304572200573)) ;
#7518=DIRECTION('ref_axis',(-0.707106781186555,-0.240631670671808,0.664903300540525)) ;
#7519=DIRECTION('',(0.,-0.940315265291054,-0.340304572200573)) ;
#7520=DIRECTION('center_axis',(1.,0.,0.)) ;
#7521=DIRECTION('ref_axis',(0.,-0.813733471206731,0.581238193719102)) ;
#7522=DIRECTION('center_axis',(0.,0.,-1.)) ;
#7523=DIRECTION('ref_axis',(-0.707106781186542,-0.707106781186553,0.)) ;
#7524=DIRECTION('',(0.,0.,-1.)) ;
#7525=DIRECTION('center_axis',(0.,0.340648777049922,-0.940190624657783)) ;
#7526=DIRECTION('ref_axis',(0.,0.940190624657783,0.340648777049922)) ;
#7527=DIRECTION('',(1.,0.,0.)) ;
#7528=DIRECTION('center_axis',(1.,0.,0.)) ;
#7529=DIRECTION('ref_axis',(0.,0.151162933346644,0.98850886064923)) ;
#7530=DIRECTION('',(1.,0.,0.)) ;
#7531=DIRECTION('center_axis',(0.,-0.504883315037953,-0.863187603129405)) ;
#7532=DIRECTION('ref_axis',(0.,0.863187603129405,-0.504883315037953)) ;
#7533=DIRECTION('',(1.,0.,0.)) ;
#7534=DIRECTION('center_axis',(1.,0.,0.)) ;
#7535=DIRECTION('ref_axis',(0.,0.977033726269219,0.213084719612847)) ;
#7536=DIRECTION('',(1.,0.,0.)) ;
#7537=DIRECTION('center_axis',(0.,-0.970879659481827,-0.239567708183828)) ;
#7538=DIRECTION('ref_axis',(0.,0.239567708183828,-0.970879659481827)) ;
#7539=DIRECTION('',(1.,0.,0.)) ;
#7540=DIRECTION('center_axis',(1.,0.,0.)) ;
#7541=DIRECTION('ref_axis',(0.,-0.970609304322144,-0.240660712130757)) ;
#7542=DIRECTION('',(1.,0.,0.)) ;
#7543=DIRECTION('center_axis',(0.,-0.707106781186548,-0.707106781186548)) ;
#7544=DIRECTION('ref_axis',(0.,0.707106781186548,-0.707106781186548)) ;
#7545=DIRECTION('',(1.,0.,0.)) ;
#7546=DIRECTION('center_axis',(1.,0.,0.)) ;
#7547=DIRECTION('ref_axis',(0.,0.999654273982356,-0.0262932027111252)) ;
#7548=DIRECTION('',(1.,0.,0.)) ;
#7549=DIRECTION('center_axis',(0.,-0.999667384056987,0.0257899447975391)) ;
#7550=DIRECTION('ref_axis',(0.,-0.0257899447975391,-0.999667384056987)) ;
#7551=DIRECTION('',(1.,0.,0.)) ;
#7552=DIRECTION('center_axis',(1.,0.,0.)) ;
#7553=DIRECTION('ref_axis',(0.,-0.649652327582147,-0.760231447170596)) ;
#7554=DIRECTION('',(1.,0.,0.)) ;
#7555=DIRECTION('center_axis',(0.,0.997575100836221,-0.0695982628490372)) ;
#7556=DIRECTION('ref_axis',(0.,0.0695982628490372,0.997575100836221)) ;
#7557=DIRECTION('',(1.,0.,0.)) ;
#7558=DIRECTION('center_axis',(0.,0.998657474351195,-0.0518000861243686)) ;
#7559=DIRECTION('ref_axis',(0.,0.0518000861243686,0.998657474351195)) ;
#7560=DIRECTION('',(1.,0.,0.)) ;
#7561=DIRECTION('center_axis',(1.,0.,0.)) ;
#7562=DIRECTION('ref_axis',(0.,0.998550602064355,-0.0538209542549495)) ;
#7563=DIRECTION('',(1.,0.,0.)) ;
#7564=DIRECTION('center_axis',(0.,0.707106781186548,0.707106781186548)) ;
#7565=DIRECTION('ref_axis',(0.,-0.707106781186548,0.707106781186548)) ;
#7566=DIRECTION('center_axis',(1.,0.,0.)) ;
#7567=DIRECTION('ref_axis',(0.,0.,-1.)) ;
#7568=DIRECTION('center_axis',(-1.,0.,0.)) ;
#7569=DIRECTION('ref_axis',(0.,0.,-1.)) ;
#7570=DIRECTION('',(0.,0.,-1.)) ;
#7571=DIRECTION('center_axis',(-1.,0.,0.)) ;
#7572=DIRECTION('ref_axis',(0.,3.41514000732436E-15,1.)) ;
#7573=DIRECTION('',(0.,0.,1.)) ;
#7574=DIRECTION('center_axis',(-1.,0.,0.)) ;
#7575=DIRECTION('ref_axis',(0.,0.,-1.)) ;
#7576=DIRECTION('center_axis',(0.,0.,-1.)) ;
#7577=DIRECTION('ref_axis',(0.707106781186548,-0.707106781186548,0.)) ;
#7578=DIRECTION('',(0.,0.,-1.)) ;
#7579=DIRECTION('center_axis',(-1.,0.,0.)) ;
#7580=DIRECTION('ref_axis',(0.,0.,1.)) ;
#7581=DIRECTION('center_axis',(-1.,0.,0.)) ;
#7582=DIRECTION('ref_axis',(0.,3.41514000732436E-15,1.)) ;
#7583=DIRECTION('center_axis',(0.,0.,1.)) ;
#7584=DIRECTION('ref_axis',(0.707106781186548,0.707106781186548,0.)) ;
#7585=DIRECTION('',(0.,0.,1.)) ;
#7586=DIRECTION('center_axis',(-1.,0.,0.)) ;
#7587=DIRECTION('ref_axis',(0.,-2.36807622294973E-14,-1.)) ;
#7588=DIRECTION('center_axis',(-1.,0.,0.)) ;
#7589=DIRECTION('ref_axis',(0.,0.,-1.)) ;
#7590=DIRECTION('center_axis',(1.,0.,0.)) ;
#7591=DIRECTION('ref_axis',(0.,-0.99972751218626,-0.0233431227103509)) ;
#7592=DIRECTION('',(1.,0.,0.)) ;
#7593=DIRECTION('center_axis',(1.,0.,0.)) ;
#7594=DIRECTION('ref_axis',(0.,0.,-1.)) ;
#7595=DIRECTION('',(1.,0.,0.)) ;
#7596=DIRECTION('center_axis',(0.,-1.,0.)) ;
#7597=DIRECTION('ref_axis',(0.,0.,-1.)) ;
#7598=DIRECTION('',(1.,0.,0.)) ;
#7599=DIRECTION('',(0.,0.,1.)) ;
#7600=DIRECTION('center_axis',(-1.,0.,0.)) ;
#7601=DIRECTION('ref_axis',(0.,0.,1.)) ;
#7602=DIRECTION('center_axis',(1.,0.,0.)) ;
#7603=DIRECTION('ref_axis',(0.,3.41514000732436E-15,1.)) ;
#7604=DIRECTION('center_axis',(-1.,0.,0.)) ;
#7605=DIRECTION('ref_axis',(0.,-3.38296603278533E-15,-1.)) ;
#7606=DIRECTION('center_axis',(0.,0.,1.)) ;
#7607=DIRECTION('ref_axis',(-0.70710678118654,0.707106781186555,0.)) ;
#7608=DIRECTION('',(0.,0.,-1.)) ;
#7609=DIRECTION('center_axis',(0.,0.,-1.)) ;
#7610=DIRECTION('ref_axis',(-0.70710678118654,-0.707106781186555,0.)) ;
#7611=DIRECTION('center_axis',(1.,0.,0.)) ;
#7612=DIRECTION('ref_axis',(0.,0.,-1.)) ;
#7613=DIRECTION('',(-1.,0.,0.)) ;
#7614=DIRECTION('center_axis',(0.,1.,0.)) ;
#7615=DIRECTION('ref_axis',(0.,0.,1.)) ;
#7616=DIRECTION('',(1.,0.,0.)) ;
#7617=DIRECTION('center_axis',(1.,0.,0.)) ;
#7618=DIRECTION('ref_axis',(0.,0.999727512186261,0.0233431227103372)) ;
#9450=CARTESIAN_POINT('',(0.,0.,0.)) ;
#9451=CARTESIAN_POINT('Origin',(-16.5,3.6,5.91295268594296)) ;
#9452=CARTESIAN_POINT('',(-16.3,3.6,19.9176877660975)) ;
#9453=CARTESIAN_POINT('',(-16.3,3.6,24.8102001714438)) ;
#9454=CARTESIAN_POINT('',(-16.3,3.6,5.91295268594296)) ;
#9455=CARTESIAN_POINT('',(-16.5,3.4,24.8)) ;
#9456=CARTESIAN_POINT('Ctrl Pts',(-16.3,3.6,24.8102001714438)) ;
#9457=CARTESIAN_POINT('Ctrl Pts',(-16.3,3.59858329627814,24.8101067420225)) ;
#9458=CARTESIAN_POINT('Ctrl Pts',(-16.3000150528782,3.59716658347763,24.8100140642958)) ;
#9459=CARTESIAN_POINT('Ctrl Pts',(-16.3005878505785,3.57021683344479,24.8082647222741)) ;
#9460=CARTESIAN_POINT('Ctrl Pts',(-16.3060170057452,3.54500851791205,24.8068523074976)) ;
#9461=CARTESIAN_POINT('Ctrl Pts',(-16.3262650142634,3.49756309113979,24.8043748002524)) ;
#9462=CARTESIAN_POINT('Ctrl Pts',(-16.3410564019887,3.47584311751711,24.8033431470145)) ;
#9463=CARTESIAN_POINT('Ctrl Pts',(-16.3781298531838,3.43929965309513,24.801671969686)) ;
#9464=CARTESIAN_POINT('Ctrl Pts',(-16.4000503702749,3.42482149959621,24.8010487344218)) ;
#9465=CARTESIAN_POINT('Ctrl Pts',(-16.4482063960532,3.40507852591201,24.8002087457528)) ;
#9466=CARTESIAN_POINT('Ctrl Pts',(-16.4739783182918,3.4,24.8)) ;
#9467=CARTESIAN_POINT('Ctrl Pts',(-16.5,3.4,24.8)) ;
#9468=CARTESIAN_POINT('',(-16.5,3.4,19.9)) ;
#9469=CARTESIAN_POINT('',(-16.5,3.4,5.91295268594296)) ;
#9470=CARTESIAN_POINT('Ctrl Pts',(-16.3,3.6,19.9176877660975)) ;
#9471=CARTESIAN_POINT('Ctrl Pts',(-16.3,3.59869799800569,19.9175543222483)) ;
#9472=CARTESIAN_POINT('Ctrl Pts',(-16.3000127140685,3.59739597782249,19.9174213564526)) ;
#9473=CARTESIAN_POINT('Ctrl Pts',(-16.3005412601056,3.57033697971358,19.9146677791384)) ;
#9474=CARTESIAN_POINT('Ctrl Pts',(-16.3060167422259,3.54489668568216,19.9122633488296)) ;
#9475=CARTESIAN_POINT('Ctrl Pts',(-16.3264311823542,3.49728852286701,19.9079677236395)) ;
#9476=CARTESIAN_POINT('Ctrl Pts',(-16.3412454459129,3.47560134784671,19.9061195584593)) ;
#9477=CARTESIAN_POINT('Ctrl Pts',(-16.3783347386739,3.43915361161839,19.90309493138)) ;
#9478=CARTESIAN_POINT('Ctrl Pts',(-16.4002305489075,3.42472405685893,19.9019445727726)) ;
#9479=CARTESIAN_POINT('Ctrl Pts',(-16.4483143342023,3.40505796847904,19.9003903114039)) ;
#9480=CARTESIAN_POINT('Ctrl Pts',(-16.4740311558542,3.4,19.9)) ;
#9481=CARTESIAN_POINT('Ctrl Pts',(-16.5,3.4,19.9)) ;
#9482=CARTESIAN_POINT('Ctrl Pts',(-16.5,3.66900151529807,25.1542076541368)) ;
#9483=CARTESIAN_POINT('Ctrl Pts',(-16.5,3.36048403150649,25.0953048518056)) ;
#9484=CARTESIAN_POINT('Ctrl Pts',(-16.5,3.40173214602619,24.7839350218989)) ;
#9485=CARTESIAN_POINT('Ctrl Pts',(-16.3,3.66900151529807,25.1542076541368)) ;
#9486=CARTESIAN_POINT('Ctrl Pts',(-16.3,3.36048403150649,25.0953048518056)) ;
#9487=CARTESIAN_POINT('Ctrl Pts',(-16.3,3.40173214602619,24.7839350218989)) ;
#9488=CARTESIAN_POINT('Ctrl Pts',(-16.3,3.70650846391527,24.9577560600852)) ;
#9489=CARTESIAN_POINT('Ctrl Pts',(-16.3,3.58356237630649,24.9342829362712)) ;
#9490=CARTESIAN_POINT('Ctrl Pts',(-16.3,3.6,24.8102001714438)) ;
#9491=CARTESIAN_POINT('',(-16.3,3.70650846391527,24.9577560600852)) ;
#9492=CARTESIAN_POINT('Origin',(-16.3,3.73135783556136,24.8276015460276)) ;
#9493=CARTESIAN_POINT('',(-16.5,3.65,25.15)) ;
#9494=CARTESIAN_POINT('Ctrl Pts',(-16.3,3.70650846391514,24.9577560600856)) ;
#9495=CARTESIAN_POINT('Ctrl Pts',(-16.3,3.70613263983865,24.9591249412769)) ;
#9496=CARTESIAN_POINT('Ctrl Pts',(-16.3000150182802,3.70575595543002,24.9604935443118)) ;
#9497=CARTESIAN_POINT('Ctrl Pts',(-16.3005875755283,3.69856163592349,24.9865707375138)) ;
#9498=CARTESIAN_POINT('Ctrl Pts',(-16.3060248879301,3.69157540066649,25.0108789195648)) ;
#9499=CARTESIAN_POINT('Ctrl Pts',(-16.3262992686171,3.67823129499146,25.0565205811117)) ;
#9500=CARTESIAN_POINT('Ctrl Pts',(-16.3410934423138,3.67201058953845,25.0773585750523)) ;
#9501=CARTESIAN_POINT('Ctrl Pts',(-16.3781678938455,3.66147275373834,25.1123866592332)) ;
#9502=CARTESIAN_POINT('Ctrl Pts',(-16.4000834311664,3.6572541549447,25.1262472800193)) ;
#9503=CARTESIAN_POINT('Ctrl Pts',(-16.4482258668633,3.6514907915847,25.1451425855636)) ;
#9504=CARTESIAN_POINT('Ctrl Pts',(-16.4739878802345,3.64999999999995,25.15)) ;
#9505=CARTESIAN_POINT('Ctrl Pts',(-16.5,3.64999999999998,25.15)) ;
#9506=CARTESIAN_POINT('Origin',(-16.5,3.73135783556136,24.8276015460276)) ;
#9507=CARTESIAN_POINT('Origin',(-16.5,9.21323262385133,26.950665756062)) ;
#9508=CARTESIAN_POINT('',(-16.3,8.97014939515602,26.862692778058)) ;
#9509=CARTESIAN_POINT('',(-16.3,9.21323262385133,26.950665756062)) ;
#9510=CARTESIAN_POINT('',(-16.5,8.9,27.05)) ;
#9511=CARTESIAN_POINT('Ctrl Pts',(-16.3,8.97014939515603,26.862692778058)) ;
#9512=CARTESIAN_POINT('Ctrl Pts',(-16.3,8.96980308364479,26.8636177522322)) ;
#9513=CARTESIAN_POINT('Ctrl Pts',(-16.3000073154306,8.96945677553284,26.8645427132193)) ;
#9514=CARTESIAN_POINT('Ctrl Pts',(-16.3004060917108,8.96001834123631,26.8897518974964)) ;
#9515=CARTESIAN_POINT('Ctrl Pts',(-16.3058295041454,8.95103756375146,26.9137357983753)) ;
#9516=CARTESIAN_POINT('Ctrl Pts',(-16.3261930199806,8.93426601854423,26.9585208446484)) ;
#9517=CARTESIAN_POINT('Ctrl Pts',(-16.3409790053634,8.92664079883567,26.9788799538846)) ;
#9518=CARTESIAN_POINT('Ctrl Pts',(-16.3780508878748,8.9138070830345,27.0131430696366)) ;
#9519=CARTESIAN_POINT('Ctrl Pts',(-16.3999818993935,8.90872114416451,27.0267199513302)) ;
#9520=CARTESIAN_POINT('Ctrl Pts',(-16.4481661967434,8.90178447987665,27.0452368074562)) ;
#9521=CARTESIAN_POINT('Ctrl Pts',(-16.4739585659257,8.90000000000001,27.05)) ;
#9522=CARTESIAN_POINT('Ctrl Pts',(-16.5,8.90000000000002,27.05)) ;
#9523=CARTESIAN_POINT('',(-16.5,9.14517170941122,27.1387288091202)) ;
#9524=CARTESIAN_POINT('Origin',(-16.5,6.94557266623349,32.0941410006498)) ;
#9525=CARTESIAN_POINT('',(-16.3,11.0061123301193,28.223872395635)) ;
#9526=CARTESIAN_POINT('Origin',(-16.3,6.94557266623349,32.0941410006498)) ;
#9527=CARTESIAN_POINT('',(-16.5,10.85,28.35)) ;
#9528=CARTESIAN_POINT('Ctrl Pts',(-16.3,11.0061123301191,28.2238723956351)) ;
#9529=CARTESIAN_POINT('Ctrl Pts',(-16.3,11.0055804043095,28.224301493411)) ;
#9530=CARTESIAN_POINT('Ctrl Pts',(-16.3000034791753,11.0050484851111,28.2247305924753)) ;
#9531=CARTESIAN_POINT('Ctrl Pts',(-16.3002811459799,10.9838233720625,28.2418531493033)) ;
#9532=CARTESIAN_POINT('Ctrl Pts',(-16.3058150165087,10.9633766729718,28.2583581483241)) ;
#9533=CARTESIAN_POINT('Ctrl Pts',(-16.326587636426,10.9257047806703,28.2887842809271)) ;
#9534=CARTESIAN_POINT('Ctrl Pts',(-16.3414529469558,10.9087812480954,28.3024612708628)) ;
#9535=CARTESIAN_POINT('Ctrl Pts',(-16.3786206798534,10.8803789404869,28.325423504731)) ;
#9536=CARTESIAN_POINT('Ctrl Pts',(-16.4005420742454,10.8691509765117,28.3345056873288)) ;
#9537=CARTESIAN_POINT('Ctrl Pts',(-16.448550854448,10.8539092421044,28.3468363151263)) ;
#9538=CARTESIAN_POINT('Ctrl Pts',(-16.4741508269864,10.85,28.35)) ;
#9539=CARTESIAN_POINT('Ctrl Pts',(-16.5,10.85,28.35)) ;
#9540=CARTESIAN_POINT('Origin',(-16.5,6.94557266623349,32.0941410006498)) ;
#9541=CARTESIAN_POINT('Origin',(-16.5,3.95376271603246,17.8309361222439)) ;
#9542=CARTESIAN_POINT('',(-16.3,11.9761936845669,29.6534659706104)) ;
#9543=CARTESIAN_POINT('',(-16.3,3.95376271603246,17.8309361222439)) ;
#9544=CARTESIAN_POINT('',(-16.5,11.8,29.75)) ;
#9545=CARTESIAN_POINT('Ctrl Pts',(-16.3,11.9761936845669,29.6534659706104)) ;
#9546=CARTESIAN_POINT('Ctrl Pts',(-16.3,11.9755977818071,29.6537918503201)) ;
#9547=CARTESIAN_POINT('Ctrl Pts',(-16.300003428101,11.9750018853708,29.6541177328253)) ;
#9548=CARTESIAN_POINT('Ctrl Pts',(-16.3002783848306,11.9511052235039,29.6671865363954)) ;
#9549=CARTESIAN_POINT('Ctrl Pts',(-16.3057856833203,11.9280772247116,29.6797901737401)) ;
#9550=CARTESIAN_POINT('Ctrl Pts',(-16.3264893687407,11.8855929764578,29.7030577904185)) ;
#9551=CARTESIAN_POINT('Ctrl Pts',(-16.3413308303542,11.866481196583,29.7135326615679)) ;
#9552=CARTESIAN_POINT('Ctrl Pts',(-16.3784493831192,11.8344052888093,29.7311205240322)) ;
#9553=CARTESIAN_POINT('Ctrl Pts',(-16.4003385455048,11.8217190498113,29.7380808841414)) ;
#9554=CARTESIAN_POINT('Ctrl Pts',(-16.4483848748457,11.8044416410206,29.7475617250063)) ;
#9555=CARTESIAN_POINT('Ctrl Pts',(-16.4740652235286,11.8,29.75)) ;
#9556=CARTESIAN_POINT('Ctrl Pts',(-16.5,11.8,29.75)) ;
#9557=CARTESIAN_POINT('',(-16.5,3.78826756115411,17.9432364059113)) ;
#9558=CARTESIAN_POINT('Origin',(-16.5,36.5141483124065,16.0157526941183)) ;
#9559=CARTESIAN_POINT('',(-16.5,23.15,2.55)) ;
#9560=CARTESIAN_POINT('',(-16.3,23.2911535787711,2.69168913909825)) ;
#9561=CARTESIAN_POINT('Ctrl Pts',(-16.5,23.15,2.55)) ;
#9562=CARTESIAN_POINT('Ctrl Pts',(-16.486729830519,23.1500114747416,2.54998861183982)) ;
#9563=CARTESIAN_POINT('Ctrl Pts',(-16.4734600075965,23.1509563633499,2.55091773409742)) ;
#9564=CARTESIAN_POINT('Ctrl Pts',(-16.4604518659889,23.1528162761338,2.55276885150634)) ;
#9565=CARTESIAN_POINT('Ctrl Pts',(-16.4474467031566,23.1546757630104,2.55461954502207)) ;
#9566=CARTESIAN_POINT('Ctrl Pts',(-16.434703780302,23.1574497571748,2.55739171292631)) ;
#9567=CARTESIAN_POINT('Ctrl Pts',(-16.4224739412131,23.1610838715948,2.56103056798632)) ;
#9568=CARTESIAN_POINT('Ctrl Pts',(-16.4102465227141,23.1647172667329,2.56466870282625)) ;
#9569=CARTESIAN_POINT('Ctrl Pts',(-16.3985326219871,23.1692102516309,2.56917299033804)) ;
#9570=CARTESIAN_POINT('Ctrl Pts',(-16.3875627358418,23.1744746360492,2.57445458125638)) ;
#9571=CARTESIAN_POINT('Ctrl Pts',(-16.3765946806012,23.1797381418269,2.57973529066242)) ;
#9572=CARTESIAN_POINT('Ctrl Pts',(-16.3663709624564,23.1857725150437,2.5857927673833)) ;
#9573=CARTESIAN_POINT('Ctrl Pts',(-16.3570926888396,23.192459275069,2.59250763886549)) ;
#9574=CARTESIAN_POINT('Ctrl Pts',(-16.3478091427317,23.1991498349263,2.59922632615453)) ;
#9575=CARTESIAN_POINT('Ctrl Pts',(-16.3394726039165,23.2064931771287,2.60660280684047)) ;
#9576=CARTESIAN_POINT('Ctrl Pts',(-16.3322472430606,23.2143449105459,2.61449159764939)) ;
#9577=CARTESIAN_POINT('Ctrl Pts',(-16.3250249191743,23.222193343716,2.62237707263526)) ;
#9578=CARTESIAN_POINT('Ctrl Pts',(-16.3189132130904,23.2305493305402,2.63077401379403)) ;
#9579=CARTESIAN_POINT('Ctrl Pts',(-16.314032381497,23.2392486759751,2.63951697966904)) ;
#9580=CARTESIAN_POINT('Ctrl Pts',(-16.3091497448563,23.2479512386341,2.6482631789001)) ;
#9581=CARTESIAN_POINT('Ctrl Pts',(-16.3054991510676,23.2569969611718,2.65735520265509)) ;
#9582=CARTESIAN_POINT('Ctrl Pts',(-16.3031524836877,23.2662079472228,2.66661380003915)) ;
#9583=CARTESIAN_POINT('Ctrl Pts',(-16.3010563665765,23.274435489668,2.67488387042443)) ;
#9584=CARTESIAN_POINT('Ctrl Pts',(-16.3,23.2827944744635,2.6832864252383)) ;
#9585=CARTESIAN_POINT('Ctrl Pts',(-16.3,23.2911535787711,2.69168913909824)) ;
#9586=CARTESIAN_POINT('',(-16.3,18.294148957922,11.4980228572171)) ;
#9587=CARTESIAN_POINT('Origin',(-16.3,36.5141483124065,16.0157526941183)) ;
#9588=CARTESIAN_POINT('',(-16.5,18.1,11.45)) ;
#9589=CARTESIAN_POINT('Ctrl Pts',(-16.3,18.2941488864465,11.4980231468811)) ;
#9590=CARTESIAN_POINT('Ctrl Pts',(-16.3,18.2931711440882,11.4977812986387)) ;
#9591=CARTESIAN_POINT('Ctrl Pts',(-16.3000076085327,18.2921934151116,11.4975394541029)) ;
#9592=CARTESIAN_POINT('Ctrl Pts',(-16.3004142507957,18.2660672742078,11.4910770538662)) ;
#9593=CARTESIAN_POINT('Ctrl Pts',(-16.3058361197429,18.2412305565793,11.4849336180022)) ;
#9594=CARTESIAN_POINT('Ctrl Pts',(-16.326188866186,18.1948292452181,11.4734561374461)) ;
#9595=CARTESIAN_POINT('Ctrl Pts',(-16.3409740368393,18.1737258010638,11.4682361612175)) ;
#9596=CARTESIAN_POINT('Ctrl Pts',(-16.3780452194892,18.1382083382951,11.459450863904)) ;
#9597=CARTESIAN_POINT('Ctrl Pts',(-16.3999768096068,18.1241338849223,11.4559695344002)) ;
#9598=CARTESIAN_POINT('Ctrl Pts',(-16.4481630630878,18.1049379542765,11.4512214053032)) ;
#9599=CARTESIAN_POINT('Ctrl Pts',(-16.4739570389763,18.0999999999998,11.4500000000009)) ;
#9600=CARTESIAN_POINT('Ctrl Pts',(-16.5,18.0999999999997,11.4500000000014)) ;
#9601=CARTESIAN_POINT('Origin',(-16.5,36.5141483124065,16.0157526941183)) ;
#9602=CARTESIAN_POINT('Origin',(-16.5,20.3521649222088,3.15764237037056)) ;
#9603=CARTESIAN_POINT('',(-16.5,16.2,19.15)) ;
#9604=CARTESIAN_POINT('',(-16.5,20.1579889903124,3.10972882873379)) ;
#9605=CARTESIAN_POINT('',(-16.3,16.39481890426,19.1953078115317)) ;
#9606=CARTESIAN_POINT('',(-16.3,20.3521649222088,3.15764237037056)) ;
#9607=CARTESIAN_POINT('Ctrl Pts',(-16.3,16.39481890426,19.1953078115317)) ;
#9608=CARTESIAN_POINT('Ctrl Pts',(-16.3,16.3937985287443,19.1950703246161)) ;
#9609=CARTESIAN_POINT('Ctrl Pts',(-16.3000082303023,16.3927781683374,19.194832844051)) ;
#9610=CARTESIAN_POINT('Ctrl Pts',(-16.3004312166973,16.3665596764086,19.1887307763087)) ;
#9611=CARTESIAN_POINT('Ctrl Pts',(-16.3058537359057,16.3416754708487,19.1829410368996)) ;
#9612=CARTESIAN_POINT('Ctrl Pts',(-16.3261949626671,16.2951486910566,19.1721187037127)) ;
#9613=CARTESIAN_POINT('Ctrl Pts',(-16.3409813386088,16.2739730545514,19.1671947135443)) ;
#9614=CARTESIAN_POINT('Ctrl Pts',(-16.3780535589099,16.2383357459206,19.1589095136144)) ;
#9615=CARTESIAN_POINT('Ctrl Pts',(-16.399984302301,16.2242141206252,19.1556273129937)) ;
#9616=CARTESIAN_POINT('Ctrl Pts',(-16.4481676790938,16.2049543635143,19.1511512193477)) ;
#9617=CARTESIAN_POINT('Ctrl Pts',(-16.4739592878869,16.2,19.15)) ;
#9618=CARTESIAN_POINT('Ctrl Pts',(-16.5,16.2,19.15)) ;
#9619=CARTESIAN_POINT('Origin',(-16.5,17.5172318824408,27.2801860892852)) ;
#9620=CARTESIAN_POINT('',(-16.3,17.1987235045029,33.2996639834704)) ;
#9621=CARTESIAN_POINT('Origin',(-16.3,17.5172318824408,27.2801860892852)) ;
#9622=CARTESIAN_POINT('',(-16.5,17.2,33.5)) ;
#9623=CARTESIAN_POINT('Ctrl Pts',(-16.3,17.1987235045029,33.2996639834704)) ;
#9624=CARTESIAN_POINT('Ctrl Pts',(-16.3,17.1987232753492,33.3003611800888)) ;
#9625=CARTESIAN_POINT('Ctrl Pts',(-16.3000036355714,17.1987230858431,33.3010583720144)) ;
#9626=CARTESIAN_POINT('Ctrl Pts',(-16.3002856442455,17.198717281846,33.328098174988)) ;
#9627=CARTESIAN_POINT('Ctrl Pts',(-16.3057480719172,17.1987708548077,33.354132367517)) ;
#9628=CARTESIAN_POINT('Ctrl Pts',(-16.3263180729416,17.1989854907429,33.4023511920969)) ;
#9629=CARTESIAN_POINT('Ctrl Pts',(-16.3411337274067,17.1991433140337,33.4241154714425)) ;
#9630=CARTESIAN_POINT('Ctrl Pts',(-16.3782330563044,17.1994835779039,33.4606980218657)) ;
#9631=CARTESIAN_POINT('Ctrl Pts',(-16.4001489369542,17.1996607382249,33.4751833159373)) ;
#9632=CARTESIAN_POINT('Ctrl Pts',(-16.448271269925,17.1999215524663,33.494923395259)) ;
#9633=CARTESIAN_POINT('Ctrl Pts',(-16.474009525343,17.2,33.5)) ;
#9634=CARTESIAN_POINT('Ctrl Pts',(-16.5,17.2,33.5)) ;
#9635=CARTESIAN_POINT('Origin',(-16.5,17.5172318824408,27.2801860892852)) ;
#9636=CARTESIAN_POINT('Origin',(-16.5,27.3698141664511,-1.38697145397653)) ;
#9637=CARTESIAN_POINT('',(-16.5,35.4,-9.7)) ;
#9638=CARTESIAN_POINT('',(-16.5,27.2283928102138,-1.52839281021384)) ;
#9639=CARTESIAN_POINT('',(-16.3,35.5417071354466,-9.55886442297199)) ;
#9640=CARTESIAN_POINT('Ctrl Pts',(-16.4999999999999,35.4,-9.70000000000001)) ;
#9641=CARTESIAN_POINT('Ctrl Pts',(-16.4867298305156,35.4000120713885,-9.7000120713885)) ;
#9642=CARTESIAN_POINT('Ctrl Pts',(-16.4734600075898,35.4009611116237,-9.69908717393026)) ;
#9643=CARTESIAN_POINT('Ctrl Pts',(-16.4604518659791,35.4028286681215,-9.69724376020955)) ;
#9644=CARTESIAN_POINT('Ctrl Pts',(-16.4474467031436,35.4046957969616,-9.69540076861792)) ;
#9645=CARTESIAN_POINT('Ctrl Pts',(-16.434703780286,35.4074809232352,-9.69263977959273)) ;
#9646=CARTESIAN_POINT('Ctrl Pts',(-16.4224739411945,35.4111294594436,-9.68901538063276)) ;
#9647=CARTESIAN_POINT('Ctrl Pts',(-16.4102465226927,35.4147772735159,-9.6853916990316)) ;
#9648=CARTESIAN_POINT('Ctrl Pts',(-16.3985326219634,35.4192879650293,-9.68090513998926)) ;
#9649=CARTESIAN_POINT('Ctrl Pts',(-16.3875627358162,35.4245730136184,-9.67564422387127)) ;
#9650=CARTESIAN_POINT('Ctrl Pts',(-16.3765946805737,35.4298571801182,-9.67038418581483)) ;
#9651=CARTESIAN_POINT('Ctrl Pts',(-16.3663709624275,35.4359151696035,-9.6643503247729)) ;
#9652=CARTESIAN_POINT('Ctrl Pts',(-16.3570926888101,35.442628054646,-9.65766156817372)) ;
#9653=CARTESIAN_POINT('Ctrl Pts',(-16.3478091427014,35.4493447543667,-9.65096901060764)) ;
#9654=CARTESIAN_POINT('Ctrl Pts',(-16.3394726038861,35.4567167467337,-9.6436211603952)) ;
#9655=CARTESIAN_POINT('Ctrl Pts',(-16.3322472430311,35.4645990935164,-9.63576295576712)) ;
#9656=CARTESIAN_POINT('Ctrl Pts',(-16.3250249191456,35.4724781271847,-9.627908054106)) ;
#9657=CARTESIAN_POINT('Ctrl Pts',(-16.3189132130632,35.4808666745071,-9.61954363879068)) ;
#9658=CARTESIAN_POINT('Ctrl Pts',(-16.3140323814724,35.4895999160555,-9.61083452924953)) ;
#9659=CARTESIAN_POINT('Ctrl Pts',(-16.3091497448343,35.4983363873636,-9.60212219887312)) ;
#9660=CARTESIAN_POINT('Ctrl Pts',(-16.3054991510491,35.5074173534341,-9.59306537373435)) ;
#9661=CARTESIAN_POINT('Ctrl Pts',(-16.3031524836736,35.5166642393525,-9.58384262874775)) ;
#9662=CARTESIAN_POINT('Ctrl Pts',(-16.3010563665718,35.524923848667,-9.57560458287265)) ;
#9663=CARTESIAN_POINT('Ctrl Pts',(-16.3,35.5333154223859,-9.56723457259326)) ;
#9664=CARTESIAN_POINT('Ctrl Pts',(-16.3,35.5417071354465,-9.55886442297206)) ;
#9665=CARTESIAN_POINT('',(-16.3,27.3698141664511,-1.38697145397653)) ;
#9666=CARTESIAN_POINT('Origin',(-16.5,17.2261159840305,33.8238840159695)) ;
#9667=CARTESIAN_POINT('',(-16.3,17.75,33.8570883563426)) ;
#9668=CARTESIAN_POINT('Origin',(-16.3,17.2261159840305,33.8238840159695)) ;
#9669=CARTESIAN_POINT('',(-16.5,17.55,33.85)) ;
#9670=CARTESIAN_POINT('Ctrl Pts',(-16.3,17.7500000000001,33.8570883563426)) ;
#9671=CARTESIAN_POINT('Ctrl Pts',(-16.3,17.7483048927982,33.8570346913121)) ;
#9672=CARTESIAN_POINT('Ctrl Pts',(-16.3000215504131,17.7466098579756,33.8569808984551)) ;
#9673=CARTESIAN_POINT('Ctrl Pts',(-16.3007065293252,17.7196757862025,33.8561240343249)) ;
#9674=CARTESIAN_POINT('Ctrl Pts',(-16.3061219364636,17.6947845328973,33.8553018126002)) ;
#9675=CARTESIAN_POINT('Ctrl Pts',(-16.3262385181079,17.6476026569698,33.8536820465369)) ;
#9676=CARTESIAN_POINT('Ctrl Pts',(-16.3410354339983,17.6258680589014,33.8529014445044)) ;
#9677=CARTESIAN_POINT('Ctrl Pts',(-16.3781172068274,17.5893078527847,33.8515452810162)) ;
#9678=CARTESIAN_POINT('Ctrl Pts',(-16.4000425477405,17.5748252688856,33.8509836241205)) ;
#9679=CARTESIAN_POINT('Ctrl Pts',(-16.4482041298703,17.555078893135,33.8502065060916)) ;
#9680=CARTESIAN_POINT('Ctrl Pts',(-16.4739769626953,17.55,33.85)) ;
#9681=CARTESIAN_POINT('Ctrl Pts',(-16.5,17.55,33.85)) ;
#9682=CARTESIAN_POINT('Origin',(-16.5,17.2261159840305,33.8238840159695)) ;
#9683=CARTESIAN_POINT('Origin',(-16.5,19.75,10.512952685943)) ;
#9684=CARTESIAN_POINT('',(-16.5,19.95,37.8)) ;
#9685=CARTESIAN_POINT('',(-16.3,19.75,37.799163194566)) ;
#9686=CARTESIAN_POINT('Ctrl Pts',(-16.5,19.95,37.8)) ;
#9687=CARTESIAN_POINT('Ctrl Pts',(-16.4867298305157,19.95,37.7999646531197)) ;
#9688=CARTESIAN_POINT('Ctrl Pts',(-16.4734600075899,19.9486749259494,37.7999293062395)) ;
#9689=CARTESIAN_POINT('Ctrl Pts',(-16.4604518659792,19.9460508737432,37.7998939593592)) ;
#9690=CARTESIAN_POINT('Ctrl Pts',(-16.4474467031437,19.9434274224269,37.7998586205732)) ;
#9691=CARTESIAN_POINT('Ctrl Pts',(-16.4347037802861,19.9395057266899,37.7998232817871)) ;
#9692=CARTESIAN_POINT('Ctrl Pts',(-16.4224739411945,19.9343629849132,37.799787943001)) ;
#9693=CARTESIAN_POINT('Ctrl Pts',(-16.4102465226928,19.9292212610131,37.7997526112094)) ;
#9694=CARTESIAN_POINT('Ctrl Pts',(-16.3985326219634,19.9228592441331,37.7997172794177)) ;
#9695=CARTESIAN_POINT('Ctrl Pts',(-16.3875627358163,19.9154021209746,37.7996819476261)) ;
#9696=CARTESIAN_POINT('Ctrl Pts',(-16.3765946805737,19.9079462424307,37.7996466217314)) ;
#9697=CARTESIAN_POINT('Ctrl Pts',(-16.3663709624276,19.8993960129258,37.7996112958368)) ;
#9698=CARTESIAN_POINT('Ctrl Pts',(-16.3570926888102,19.8899196212419,37.7995759699421)) ;
#9699=CARTESIAN_POINT('Ctrl Pts',(-16.3478091427015,19.8804378444838,37.7995406239731)) ;
#9700=CARTESIAN_POINT('Ctrl Pts',(-16.3394726038862,19.8700293439778,37.7995052780041)) ;
#9701=CARTESIAN_POINT('Ctrl Pts',(-16.3322472430311,19.8588990933357,37.799469932035)) ;
#9702=CARTESIAN_POINT('Ctrl Pts',(-16.3250249191456,19.8477735209695,37.7994346009226)) ;
#9703=CARTESIAN_POINT('Ctrl Pts',(-16.3189132130633,19.8359273874834,37.7993992698103)) ;
#9704=CARTESIAN_POINT('Ctrl Pts',(-16.3140323814724,19.8235937827482,37.7993639386979)) ;
#9705=CARTESIAN_POINT('Ctrl Pts',(-16.3091497448343,19.8112556167534,37.7993285945192)) ;
#9706=CARTESIAN_POINT('Ctrl Pts',(-16.3054991510491,19.7984302615936,37.7992932503405)) ;
#9707=CARTESIAN_POINT('Ctrl Pts',(-16.3031524836737,19.7853702603347,37.7992579061619)) ;
#9708=CARTESIAN_POINT('Ctrl Pts',(-16.3010563665718,19.7737046564764,37.7992263356299)) ;
#9709=CARTESIAN_POINT('Ctrl Pts',(-16.3,19.7618524267677,37.799194765098)) ;
#9710=CARTESIAN_POINT('Ctrl Pts',(-16.3,19.75,37.799163194566)) ;
#9711=CARTESIAN_POINT('',(-16.3,19.75,33.9947419676036)) ;
#9712=CARTESIAN_POINT('',(-16.3,19.75,10.512952685943)) ;
#9713=CARTESIAN_POINT('',(-16.5,19.95,34.)) ;
#9714=CARTESIAN_POINT('Ctrl Pts',(-16.3,19.75,33.9947419676036)) ;
#9715=CARTESIAN_POINT('Ctrl Pts',(-16.3,19.7510782785912,33.9947695469051)) ;
#9716=CARTESIAN_POINT('Ctrl Pts',(-16.3000087201354,19.7521565392984,33.9947971375259)) ;
#9717=CARTESIAN_POINT('Ctrl Pts',(-16.3002171823642,19.7650440705554,33.9951270456112)) ;
#9718=CARTESIAN_POINT('Ctrl Pts',(-16.3014539310975,19.7768134007127,33.9954297554171)) ;
#9719=CARTESIAN_POINT('Ctrl Pts',(-16.3063661361484,19.8019186718149,33.9960784841571)) ;
#9720=CARTESIAN_POINT('Ctrl Pts',(-16.3103990384751,19.8151237982275,33.9964216349601)) ;
#9721=CARTESIAN_POINT('Ctrl Pts',(-16.3258880628794,19.8517998580413,33.9973795771215)) ;
#9722=CARTESIAN_POINT('Ctrl Pts',(-16.3406089202894,19.8735832081072,33.9979548913887)) ;
#9723=CARTESIAN_POINT('Ctrl Pts',(-16.3775678942223,19.9102753697401,33.9989306239122)) ;
#9724=CARTESIAN_POINT('Ctrl Pts',(-16.3994500653805,19.9248361652066,33.9993215857928)) ;
#9725=CARTESIAN_POINT('Ctrl Pts',(-16.4475619545613,19.9447510071692,33.9998577643717)) ;
#9726=CARTESIAN_POINT('Ctrl Pts',(-16.473330252482,19.9499162250234,33.9999977343853)) ;
#9727=CARTESIAN_POINT('Ctrl Pts',(-16.4995761386499,19.9499996631663,33.9999999908907)) ;
#9728=CARTESIAN_POINT('Ctrl Pts',(-16.4997880774491,19.95,34.)) ;
#9729=CARTESIAN_POINT('Ctrl Pts',(-16.5,19.95,34.)) ;
#9730=CARTESIAN_POINT('',(-16.5,19.95,10.512952685943)) ;
#9731=CARTESIAN_POINT('Origin',(-16.5,43.2596418025572,-36.388001295162)) ;
#9732=CARTESIAN_POINT('',(-16.5,42.3,-58.75)) ;
#9733=CARTESIAN_POINT('',(-16.5,44.45,-17.3)) ;
#9734=CARTESIAN_POINT('',(-16.5,43.4593732974275,-36.3983613123869)) ;
#9735=CARTESIAN_POINT('',(-16.3,44.2502789878669,-17.2894378853552)) ;
#9736=CARTESIAN_POINT('Ctrl Pts',(-16.5000000000003,44.45,-17.3)) ;
#9737=CARTESIAN_POINT('Ctrl Pts',(-16.4867298305159,44.4500004427936,-17.2999914633522)) ;
#9738=CARTESIAN_POINT('Ctrl Pts',(-16.4734600075901,44.4486775904825,-17.2999142877544)) ;
#9739=CARTESIAN_POINT('Ctrl Pts',(-16.4604518659795,44.4460575039272,-17.2997698249763)) ;
#9740=CARTESIAN_POINT('Ctrl Pts',(-16.447446703144,44.4434380173538,-17.2996253952791)) ;
#9741=CARTESIAN_POINT('Ctrl Pts',(-16.4347037802864,44.439522029286,-17.2994137164092)) ;
#9742=CARTESIAN_POINT('Ctrl Pts',(-16.4224739411948,44.4343866344642,-17.2991387872492)) ;
#9743=CARTESIAN_POINT('Ctrl Pts',(-16.410246522693,44.429252256065,-17.2988639125046)) ;
#9744=CARTESIAN_POINT('Ctrl Pts',(-16.3985326219637,44.4228992229604,-17.2985258264785)) ;
#9745=CARTESIAN_POINT('Ctrl Pts',(-16.3875627358166,44.4154525537855,-17.2981310138529)) ;
#9746=CARTESIAN_POINT('Ctrl Pts',(-16.376594680574,44.4080071274804,-17.2977362671226)) ;
#9747=CARTESIAN_POINT('Ctrl Pts',(-16.3663709624278,44.3994688194087,-17.2972848329182)) ;
#9748=CARTESIAN_POINT('Ctrl Pts',(-16.3570926888104,44.3900055925544,-17.2967854234333)) ;
#9749=CARTESIAN_POINT('Ctrl Pts',(-16.3478091427017,44.3805369881069,-17.2962857301528)) ;
#9750=CARTESIAN_POINT('Ctrl Pts',(-16.3394726038863,44.370142904062,-17.2957380325024)) ;
#9751=CARTESIAN_POINT('Ctrl Pts',(-16.3322472430313,44.3590280388489,-17.2951529481328)) ;
#9752=CARTESIAN_POINT('Ctrl Pts',(-16.3250249191457,44.3479178454451,-17.2945681096863)) ;
#9753=CARTESIAN_POINT('Ctrl Pts',(-16.3189132130634,44.336088058293,-17.2939459461117)) ;
#9754=CARTESIAN_POINT('Ctrl Pts',(-16.3140323814725,44.3237714543345,-17.2932985314845)) ;
#9755=CARTESIAN_POINT('Ctrl Pts',(-16.3091497448344,44.3114502954038,-17.292650877428)) ;
#9756=CARTESIAN_POINT('Ctrl Pts',(-16.3054991510492,44.298642601372,-17.2919779869307)) ;
#9757=CARTESIAN_POINT('Ctrl Pts',(-16.3031524836737,44.2856005762595,-17.2912929417453)) ;
#9758=CARTESIAN_POINT('Ctrl Pts',(-16.3010563665718,44.2739510292602,-17.2906810378413)) ;
#9759=CARTESIAN_POINT('Ctrl Pts',(-16.3,44.2621151069607,-17.290059466702)) ;
#9760=CARTESIAN_POINT('Ctrl Pts',(-16.3,44.2502789878666,-17.2894378853551)) ;
#9761=CARTESIAN_POINT('',(-16.3,42.1003608836993,-58.737859058676)) ;
#9762=CARTESIAN_POINT('',(-16.3,43.2596418025572,-36.388001295162)) ;
#9763=CARTESIAN_POINT('Origin',(-16.5,42.1003608738345,-58.7378592000713)) ;
#9764=CARTESIAN_POINT('Origin',(-16.5,21.6437725346931,34.0916800205589)) ;
#9765=CARTESIAN_POINT('',(-16.3,20.6462198057265,32.4790238413936)) ;
#9766=CARTESIAN_POINT('Origin',(-16.3,21.6437725346931,34.0916800205589)) ;
#9767=CARTESIAN_POINT('',(-16.5,20.75,32.65)) ;
#9768=CARTESIAN_POINT('Ctrl Pts',(-16.3,20.6462198057265,32.4790238413936)) ;
#9769=CARTESIAN_POINT('Ctrl Pts',(-16.3,20.6471046707134,32.4804826685849)) ;
#9770=CARTESIAN_POINT('Ctrl Pts',(-16.3000218320537,20.6479895107055,32.4819414292721)) ;
#9771=CARTESIAN_POINT('Ctrl Pts',(-16.3007104860663,20.661942770123,32.5049445855192)) ;
#9772=CARTESIAN_POINT('Ctrl Pts',(-16.3061131716744,20.67483374418,32.5261907507504)) ;
#9773=CARTESIAN_POINT('Ctrl Pts',(-16.3261915748286,20.6992980016081,32.5665017177397)) ;
#9774=CARTESIAN_POINT('Ctrl Pts',(-16.3409772878684,20.7105794706497,32.58508542171)) ;
#9775=CARTESIAN_POINT('Ctrl Pts',(-16.3780489386812,20.7295683313049,32.6163598571282)) ;
#9776=CARTESIAN_POINT('Ctrl Pts',(-16.3999801547909,20.737094268172,32.6287518987764)) ;
#9777=CARTESIAN_POINT('Ctrl Pts',(-16.4481651260864,20.7473591549605,32.6456526692713)) ;
#9778=CARTESIAN_POINT('Ctrl Pts',(-16.4739580437547,20.75,32.65)) ;
#9779=CARTESIAN_POINT('Ctrl Pts',(-16.5,20.75,32.65)) ;
#9780=CARTESIAN_POINT('Origin',(-16.5,21.6437725346931,34.0916800205589)) ;
#9781=CARTESIAN_POINT('Origin',(-16.5,23.7122919887408,-16.1822567109578)) ;
#9782=CARTESIAN_POINT('',(-16.5,38.35,-1.45)) ;
#9783=CARTESIAN_POINT('Origin',(-16.5,23.7122919887408,-16.1822567109578)) ;
#9784=CARTESIAN_POINT('',(-16.3,38.2088062759988,-1.59164899203244)) ;
#9785=CARTESIAN_POINT('Ctrl Pts',(-16.5,38.35,-1.45)) ;
#9786=CARTESIAN_POINT('Ctrl Pts',(-16.4867298305176,38.3499902600277,-1.44999032253691)) ;
#9787=CARTESIAN_POINT('Ctrl Pts',(-16.4734600075938,38.3490465723702,-1.4509206253905)) ;
#9788=CARTESIAN_POINT('Ctrl Pts',(-16.4604518659851,38.3471873356328,-1.45277240215352)) ;
#9789=CARTESIAN_POINT('Ctrl Pts',(-16.4474467031515,38.3453285246479,-1.45462375487236)) ;
#9790=CARTESIAN_POINT('Ctrl Pts',(-16.4347037802957,38.3425546817605,-1.45739606102526)) ;
#9791=CARTESIAN_POINT('Ctrl Pts',(-16.4224739412057,38.3389202236103,-1.46103456278714)) ;
#9792=CARTESIAN_POINT('Ctrl Pts',(-16.4102465227056,38.33528648481,-1.46467234439889)) ;
#9793=CARTESIAN_POINT('Ctrl Pts',(-16.3985326219777,38.3307926615411,-1.46917578743196)) ;
#9794=CARTESIAN_POINT('Ctrl Pts',(-16.3875627358317,38.3255269931887,-1.47445609142917)) ;
#9795=CARTESIAN_POINT('Ctrl Pts',(-16.3765946805903,38.320262203691,-1.4797355141289)) ;
#9796=CARTESIAN_POINT('Ctrl Pts',(-16.3663709624449,38.3142261014913,-1.48579126199939)) ;
#9797=CARTESIAN_POINT('Ctrl Pts',(-16.3570926888279,38.3075372339825,-1.49250402878747)) ;
#9798=CARTESIAN_POINT('Ctrl Pts',(-16.3478091427197,38.3008445654438,-1.49922061018643)) ;
#9799=CARTESIAN_POINT('Ctrl Pts',(-16.3394726039044,38.2934987358228,-1.5065946089037)) ;
#9800=CARTESIAN_POINT('Ctrl Pts',(-16.3322472430489,38.2856442181935,-1.51448062303995)) ;
#9801=CARTESIAN_POINT('Ctrl Pts',(-16.3250249191629,38.2777930019814,-1.52236332252028)) ;
#9802=CARTESIAN_POINT('Ctrl Pts',(-16.3189132130796,38.2694339358032,-1.53075719394756)) ;
#9803=CARTESIAN_POINT('Ctrl Pts',(-16.3140323814872,38.2607313083892,-1.5394968888988)) ;
#9804=CARTESIAN_POINT('Ctrl Pts',(-16.3091497448476,38.2520254625372,-1.54823981599646)) ;
#9805=CARTESIAN_POINT('Ctrl Pts',(-16.3054991510602,38.2429762542893,-1.55732836653302)) ;
#9806=CARTESIAN_POINT('Ctrl Pts',(-16.3031524836821,38.233761681978,-1.56658339086779)) ;
#9807=CARTESIAN_POINT('Ctrl Pts',(-16.3010563665746,38.2255309361809,-1.57485026968463)) ;
#9808=CARTESIAN_POINT('Ctrl Pts',(-16.3,38.2171686680524,-1.58324955352066)) ;
#9809=CARTESIAN_POINT('Ctrl Pts',(-16.3,38.2088062759988,-1.59164899203244)) ;
#9810=CARTESIAN_POINT('Origin',(-16.3,23.7122919887408,-16.1822567109578)) ;
#9811=CARTESIAN_POINT('Origin',(-16.5,17.453364864871,27.1098816953352)) ;
#9812=CARTESIAN_POINT('',(-16.3,23.7,27.1493776981789)) ;
#9813=CARTESIAN_POINT('Origin',(-16.3,17.453364864871,27.1098816953352)) ;
#9814=CARTESIAN_POINT('',(-16.5,23.9,27.15)) ;
#9815=CARTESIAN_POINT('Ctrl Pts',(-16.3,23.7000000155168,27.1493727892874)) ;
#9816=CARTESIAN_POINT('Ctrl Pts',(-16.3000000001223,23.701576033318,27.1493777710131)) ;
#9817=CARTESIAN_POINT('Ctrl Pts',(-16.300018628741,23.7031519805708,27.1493827515887)) ;
#9818=CARTESIAN_POINT('Ctrl Pts',(-16.3006547601165,23.7300560874974,27.1494677621026)) ;
#9819=CARTESIAN_POINT('Ctrl Pts',(-16.3060610729129,23.7550416808744,27.1495464596783)) ;
#9820=CARTESIAN_POINT('Ctrl Pts',(-16.3261891818602,23.8023134117509,27.1496949552357)) ;
#9821=CARTESIAN_POINT('Ctrl Pts',(-16.3409744121654,23.8240528090639,27.1497630282075)) ;
#9822=CARTESIAN_POINT('Ctrl Pts',(-16.3780456454816,23.8606404855451,27.149877384696)) ;
#9823=CARTESIAN_POINT('Ctrl Pts',(-16.3999771910801,23.8751390022259,27.1499225811532)) ;
#9824=CARTESIAN_POINT('Ctrl Pts',(-16.4481632972522,23.8949132761296,27.1499841811634)) ;
#9825=CARTESIAN_POINT('Ctrl Pts',(-16.4739571531563,23.9,27.15)) ;
#9826=CARTESIAN_POINT('Ctrl Pts',(-16.5,23.9,27.15)) ;
#9827=CARTESIAN_POINT('Origin',(-16.5,17.453364864871,27.1098816953352)) ;
#9828=CARTESIAN_POINT('Origin',(-16.5,33.4726637867458,16.9651420152427)) ;
#9829=CARTESIAN_POINT('',(-16.5,23.9,16.95)) ;
#9830=CARTESIAN_POINT('',(-16.3,23.7000000012803,16.9498418202582)) ;
#9831=CARTESIAN_POINT('Ctrl Pts',(-16.5,23.9,16.95)) ;
#9832=CARTESIAN_POINT('Ctrl Pts',(-16.4867298305178,23.8999999896474,16.950006544798)) ;
#9833=CARTESIAN_POINT('Ctrl Pts',(-16.4734600075941,23.8986749069092,16.9500109936177)) ;
#9834=CARTESIAN_POINT('Ctrl Pts',(-16.4604518659855,23.8960508476347,16.950013395784)) ;
#9835=CARTESIAN_POINT('Ctrl Pts',(-16.447446703152,23.8934273892517,16.9500157974002)) ;
#9836=CARTESIAN_POINT('Ctrl Pts',(-16.4347037802963,23.8895056880666,16.9500161535546)) ;
#9837=CARTESIAN_POINT('Ctrl Pts',(-16.4224739412065,23.8843629423518,16.9500145938707)) ;
#9838=CARTESIAN_POINT('Ctrl Pts',(-16.4102465227065,23.8792212145144,16.9500130344956)) ;
#9839=CARTESIAN_POINT('Ctrl Pts',(-16.3985326219787,23.8728591952062,16.9500095604991)) ;
#9840=CARTESIAN_POINT('Ctrl Pts',(-16.3875627358327,23.8654020709616,16.9500043763796)) ;
#9841=CARTESIAN_POINT('Ctrl Pts',(-16.3765946805914,23.8579461913319,16.9499991931253)) ;
#9842=CARTESIAN_POINT('Ctrl Pts',(-16.3663709624461,23.8493959620825,16.9499923009626)) ;
#9843=CARTESIAN_POINT('Ctrl Pts',(-16.3570926888291,23.839919571777,16.9499839709371)) ;
#9844=CARTESIAN_POINT('Ctrl Pts',(-16.347809142721,23.8304377963981,16.9499756361781)) ;
#9845=CARTESIAN_POINT('Ctrl Pts',(-16.3394726039057,23.820029298395,16.9499658627199)) ;
#9846=CARTESIAN_POINT('Ctrl Pts',(-16.3322472430501,23.8088990511176,16.9499549779694)) ;
#9847=CARTESIAN_POINT('Ctrl Pts',(-16.3250249191641,23.797773482115,16.9499440977939)) ;
#9848=CARTESIAN_POINT('Ctrl Pts',(-16.3189132130807,23.7859273528529,16.9499321081945)) ;
#9849=CARTESIAN_POINT('Ctrl Pts',(-16.3140323814882,23.7735937529089,16.949919378958)) ;
#9850=CARTESIAN_POINT('Ctrl Pts',(-16.3091497448485,23.7612555917073,16.9499066450139)) ;
#9851=CARTESIAN_POINT('Ctrl Pts',(-16.305499151061,23.7484302419074,16.9498931719074)) ;
#9852=CARTESIAN_POINT('Ctrl Pts',(-16.3031524836827,23.735370246261,16.9498793579648)) ;
#9853=CARTESIAN_POINT('Ctrl Pts',(-16.3010563665748,23.7237046473967,16.9498670189167)) ;
#9854=CARTESIAN_POINT('Ctrl Pts',(-16.3,23.7118524228822,16.9498544088282)) ;
#9855=CARTESIAN_POINT('Ctrl Pts',(-16.3,23.7000000012803,16.9498418202582)) ;
#9856=CARTESIAN_POINT('',(-16.3,26.5585000901577,10.0586572410252)) ;
#9857=CARTESIAN_POINT('Origin',(-16.3,33.4726637867458,16.9651420152427)) ;
#9858=CARTESIAN_POINT('',(-16.5,26.7,10.2)) ;
#9859=CARTESIAN_POINT('Origin',(-16.5,26.5585000901577,10.0586572410252)) ;
#9860=CARTESIAN_POINT('Origin',(-16.5,33.4726637867458,16.9651420152427)) ;
#9861=CARTESIAN_POINT('Origin',(-16.5,23.7,1.98795268594296)) ;
#9862=CARTESIAN_POINT('',(-16.3,23.7,1.98795268594296)) ;
#9863=CARTESIAN_POINT('',(-16.5,23.9,1.98795268594296)) ;
#9864=CARTESIAN_POINT('Origin',(-16.5,37.4869714539765,-0.869814166451151)) ;
#9865=CARTESIAN_POINT('',(-16.5,37.6283928102138,-0.72839281021384)) ;
#9866=CARTESIAN_POINT('',(-16.3,37.4869714539765,-0.869814166451151)) ;
#9867=CARTESIAN_POINT('Origin',(-16.5,43.5701155187154,-37.6713759567788)) ;
#9868=CARTESIAN_POINT('',(-16.5,42.15,-60.9)) ;
#9869=CARTESIAN_POINT('',(-16.5,43.7696305388826,-37.6852956093486)) ;
#9870=CARTESIAN_POINT('',(-16.3,41.9506268879594,-60.8840463309467)) ;
#9871=CARTESIAN_POINT('',(-16.3,43.5701155187154,-37.6713759567788)) ;
#9872=CARTESIAN_POINT('Ctrl Pts',(-16.3,41.9506268879594,-60.8840463309467)) ;
#9873=CARTESIAN_POINT('Ctrl Pts',(-16.3,41.9517471911502,-60.8841361107774)) ;
#9874=CARTESIAN_POINT('Ctrl Pts',(-16.3000094725398,41.9528674746344,-60.8842258867201)) ;
#9875=CARTESIAN_POINT('Ctrl Pts',(-16.3004632147513,41.9796968069122,-60.8863758482814)) ;
#9876=CARTESIAN_POINT('Ctrl Pts',(-16.3058831665225,42.0050812395992,-60.8884087660428)) ;
#9877=CARTESIAN_POINT('Ctrl Pts',(-16.3261922917654,42.0526243758533,-60.8922143172951)) ;
#9878=CARTESIAN_POINT('Ctrl Pts',(-16.3409781044896,42.074295218724,-60.893947902738)) ;
#9879=CARTESIAN_POINT('Ctrl Pts',(-16.3780498309033,42.1107665799089,-60.8968644715331)) ;
#9880=CARTESIAN_POINT('Ctrl Pts',(-16.3999809367931,42.1252187814051,-60.8980196294309)) ;
#9881=CARTESIAN_POINT('Ctrl Pts',(-16.4481655949025,42.1449296139692,-60.8995949062458)) ;
#9882=CARTESIAN_POINT('Ctrl Pts',(-16.4739582736902,42.15,-60.8999999999999)) ;
#9883=CARTESIAN_POINT('Ctrl Pts',(-16.5,42.1500000000001,-60.8999999999991)) ;
#9884=CARTESIAN_POINT('Origin',(-16.5,18.75,37.7899579831933)) ;
#9885=CARTESIAN_POINT('',(-16.5,17.55,37.8)) ;
#9886=CARTESIAN_POINT('',(-16.3,17.7500003499425,37.7991631591148)) ;
#9887=CARTESIAN_POINT('Ctrl Pts',(-16.5,17.55,37.8)) ;
#9888=CARTESIAN_POINT('Ctrl Pts',(-16.4867298362033,17.5500003549376,37.8000424142976)) ;
#9889=CARTESIAN_POINT('Ctrl Pts',(-16.4734600189644,17.55132573864,37.8000737393719)) ;
#9890=CARTESIAN_POINT('Ctrl Pts',(-16.4604518827053,17.5539500526455,37.8000937776279)) ;
#9891=CARTESIAN_POINT('Ctrl Pts',(-16.4474467253984,17.5565737656652,37.8001138112951)) ;
#9892=CARTESIAN_POINT('Ctrl Pts',(-16.4347038077254,17.5604956752289,37.8001225626839)) ;
#9893=CARTESIAN_POINT('Ctrl Pts',(-16.4224739731519,17.5656385824154,37.8001202894756)) ;
#9894=CARTESIAN_POINT('Ctrl Pts',(-16.4102465594111,17.57078047159,37.8001180167172)) ;
#9895=CARTESIAN_POINT('Ctrl Pts',(-16.3985326627544,17.5771426052934,37.8001047243444)) ;
#9896=CARTESIAN_POINT('Ctrl Pts',(-16.3875627796997,17.584599798429,37.8000811250022)) ;
#9897=CARTESIAN_POINT('Ctrl Pts',(-16.3765947278103,17.5920557467608,37.8000575295993)) ;
#9898=CARTESIAN_POINT('Ctrl Pts',(-16.3663710120005,17.600605999172,37.8000236325339)) ;
#9899=CARTESIAN_POINT('Ctrl Pts',(-16.3570927394624,17.6100823706619,37.7999805824503)) ;
#9900=CARTESIAN_POINT('Ctrl Pts',(-16.3478091947644,17.6195641268768,37.7999375079045)) ;
#9901=CARTESIAN_POINT('Ctrl Pts',(-16.3394726560326,17.6299725636313,37.7998852729588)) ;
#9902=CARTESIAN_POINT('Ctrl Pts',(-16.3322472937619,17.6411027132277,37.7998254284371)) ;
#9903=CARTESIAN_POINT('Ctrl Pts',(-16.3250249685983,17.6522281843796,37.7997656090704)) ;
#9904=CARTESIAN_POINT('Ctrl Pts',(-16.3189132596971,17.6640741793753,37.7996981907095)) ;
#9905=CARTESIAN_POINT('Ctrl Pts',(-16.3140324236727,17.6764076162048,37.7996250677075)) ;
#9906=CARTESIAN_POINT('Ctrl Pts',(-16.3091497826833,17.6887456140198,37.7995519176641)) ;
#9907=CARTESIAN_POINT('Ctrl Pts',(-16.3054991828882,17.7015707715661,37.7994730638621)) ;
#9908=CARTESIAN_POINT('Ctrl Pts',(-16.3031525078829,17.7146305553493,37.7993906788029)) ;
#9909=CARTESIAN_POINT('Ctrl Pts',(-16.3010563747267,17.7262960163692,37.7993170895528)) ;
#9910=CARTESIAN_POINT('Ctrl Pts',(-16.3,17.7381480890742,37.7992406894262)) ;
#9911=CARTESIAN_POINT('Ctrl Pts',(-16.3,17.7500003499425,37.7991631591148)) ;
#9912=CARTESIAN_POINT('Origin',(-16.3,18.75,37.7899579831933)) ;
#9913=CARTESIAN_POINT('Origin',(-16.5,18.75,37.7899579831933)) ;
#9914=CARTESIAN_POINT('Origin',(-16.5,37.7318176617063,-60.502128268216)) ;
#9915=CARTESIAN_POINT('',(-16.5,36.65,-56.2)) ;
#9916=CARTESIAN_POINT('Origin',(-16.5,37.7318176617063,-60.502128268216)) ;
#9917=CARTESIAN_POINT('',(-16.3,36.8459456848986,-56.3597323992937)) ;
#9918=CARTESIAN_POINT('Origin',(-16.3,37.7318176617063,-60.502128268216)) ;
#9919=CARTESIAN_POINT('Ctrl Pts',(-16.3,36.8459456848986,-56.3597323992937)) ;
#9920=CARTESIAN_POINT('Ctrl Pts',(-16.3,36.8452932432187,-56.3591906677183)) ;
#9921=CARTESIAN_POINT('Ctrl Pts',(-16.3000033286272,36.8446407490739,-56.3586489949852)) ;
#9922=CARTESIAN_POINT('Ctrl Pts',(-16.3001926160016,36.8260916784102,-56.3432532583223)) ;
#9923=CARTESIAN_POINT('Ctrl Pts',(-16.3028806855463,36.8081301664174,-56.328423604229)) ;
#9924=CARTESIAN_POINT('Ctrl Pts',(-16.3132358643299,36.7736693811157,-56.3001110660322)) ;
#9925=CARTESIAN_POINT('Ctrl Pts',(-16.3207681279902,36.7570768798036,-56.2865472202179)) ;
#9926=CARTESIAN_POINT('Ctrl Pts',(-16.3435477982502,36.7216811428078,-56.2577328860845)) ;
#9927=CARTESIAN_POINT('Ctrl Pts',(-16.3603327562665,36.7034378018957,-56.2429732328781)) ;
#9928=CARTESIAN_POINT('Ctrl Pts',(-16.3980903936837,36.6760935350204,-56.220928962173)) ;
#9929=CARTESIAN_POINT('Ctrl Pts',(-16.417515115282,36.6660883821569,-56.2128959810192)) ;
#9930=CARTESIAN_POINT('Ctrl Pts',(-16.4584357635178,36.653234532305,-56.2025876834372)) ;
#9931=CARTESIAN_POINT('Ctrl Pts',(-16.4790164237796,36.65,-56.2)) ;
#9932=CARTESIAN_POINT('Ctrl Pts',(-16.5,36.65,-56.2)) ;
#9933=CARTESIAN_POINT('Origin',(-16.5,17.75,12.412952685943)) ;
#9934=CARTESIAN_POINT('',(-16.3,17.75,12.412952685943)) ;
#9935=CARTESIAN_POINT('',(-16.5,17.55,12.412952685943)) ;
#9936=CARTESIAN_POINT('Origin',(-16.5,29.7633733578399,-15.291248496029)) ;
#9937=CARTESIAN_POINT('',(-16.5,37.7,-15.5)) ;
#9938=CARTESIAN_POINT('Origin',(-16.5,29.7633733578399,-15.291248496029)) ;
#9939=CARTESIAN_POINT('',(-16.3,37.8999308547965,-15.5052586405422)) ;
#9940=CARTESIAN_POINT('Origin',(-16.5,37.8999308547965,-15.5052586405422)) ;
#9941=CARTESIAN_POINT('Origin',(-16.3,29.7633733578399,-15.291248496029)) ;
#9942=CARTESIAN_POINT('Origin',(-16.5,37.9279179147939,-14.4204278690655)) ;
#9943=CARTESIAN_POINT('',(-16.3,37.9279179147939,-14.4204278690655)) ;
#9944=CARTESIAN_POINT('',(-16.5,37.7279844379825,-14.415269880106)) ;
#9945=CARTESIAN_POINT('Origin',(-16.5,12.5256959686759,18.3486581187154)) ;
#9946=CARTESIAN_POINT('',(-16.5,15.5,20.65)) ;
#9947=CARTESIAN_POINT('Origin',(-16.5,12.5256959686759,18.3486581187154)) ;
#9948=CARTESIAN_POINT('',(-16.3,15.63399980594,20.8033220974013)) ;
#9949=CARTESIAN_POINT('Origin',(-16.3,12.5256959686759,18.3486581187154)) ;
#9950=CARTESIAN_POINT('Ctrl Pts',(-16.3,15.63399980594,20.8033220974013)) ;
#9951=CARTESIAN_POINT('Ctrl Pts',(-16.3,15.6335509952834,20.8028060276236)) ;
#9952=CARTESIAN_POINT('Ctrl Pts',(-16.3000033875055,15.633102174688,20.8022899714548)) ;
#9953=CARTESIAN_POINT('Ctrl Pts',(-16.300280172625,15.6147658776647,20.7812078286703)) ;
#9954=CARTESIAN_POINT('Ctrl Pts',(-16.3059282130228,15.5970507182787,20.7608811682357)) ;
#9955=CARTESIAN_POINT('Ctrl Pts',(-16.3270273887872,15.5646346653857,20.7237524476597)) ;
#9956=CARTESIAN_POINT('Ctrl Pts',(-16.341968842749,15.5501345809321,20.7071773901075)) ;
#9957=CARTESIAN_POINT('Ctrl Pts',(-16.3791047732673,15.5259533953226,20.6795690847363)) ;
#9958=CARTESIAN_POINT('Ctrl Pts',(-16.4008132433006,15.5164134390286,20.6686952926497)) ;
#9959=CARTESIAN_POINT('Ctrl Pts',(-16.448352927527,15.5034318834199,20.6539056000502)) ;
#9960=CARTESIAN_POINT('Ctrl Pts',(-16.4736593458904,15.500064924654,20.6500739112853)) ;
#9961=CARTESIAN_POINT('Ctrl Pts',(-16.4995041564433,15.5000003098668,20.6500003527573)) ;
#9962=CARTESIAN_POINT('Ctrl Pts',(-16.4997520907635,15.5,20.65)) ;
#9963=CARTESIAN_POINT('Ctrl Pts',(-16.5,15.5,20.65)) ;
#9964=CARTESIAN_POINT('Origin',(-16.5,24.7469152941988,15.4731262457782)) ;
#9965=CARTESIAN_POINT('',(-16.5,12.85,22.2)) ;
#9966=CARTESIAN_POINT('',(-16.5,24.6459386311912,15.3004887251523)) ;
#9967=CARTESIAN_POINT('',(-16.3,12.9183976933795,22.3916931443706)) ;
#9968=CARTESIAN_POINT('',(-16.3,24.7469152941988,15.4731262457782)) ;
#9969=CARTESIAN_POINT('Ctrl Pts',(-16.3,12.9183976933795,22.3916931443706)) ;
#9970=CARTESIAN_POINT('Ctrl Pts',(-16.3,12.9181668378952,22.3910505718131)) ;
#9971=CARTESIAN_POINT('Ctrl Pts',(-16.3000033789794,12.9179359974519,22.3904079978298)) ;
#9972=CARTESIAN_POINT('Ctrl Pts',(-16.30027972266,12.9084972701201,22.3641323186868)) ;
#9973=CARTESIAN_POINT('Ctrl Pts',(-16.3059239690591,12.8994116223236,22.3387679571224)) ;
#9974=CARTESIAN_POINT('Ctrl Pts',(-16.3270129833413,12.8828359249044,22.2923792487433)) ;
#9975=CARTESIAN_POINT('Ctrl Pts',(-16.3419513881418,12.8754470934585,22.2716433563484)) ;
#9976=CARTESIAN_POINT('Ctrl Pts',(-16.3790879803581,12.8631486026243,22.2370711958976)) ;
#9977=CARTESIAN_POINT('Ctrl Pts',(-16.4008036126822,12.8583107467619,22.2234396941227)) ;
#9978=CARTESIAN_POINT('Ctrl Pts',(-16.4483630640904,12.8517330735393,22.2048939197986)) ;
#9979=CARTESIAN_POINT('Ctrl Pts',(-16.4736838335087,12.8500311854431,22.2000880211873)) ;
#9980=CARTESIAN_POINT('Ctrl Pts',(-16.4995289737795,12.8500001414228,22.2000003991673)) ;
#9981=CARTESIAN_POINT('Ctrl Pts',(-16.4997644981787,12.85,22.2)) ;
#9982=CARTESIAN_POINT('Ctrl Pts',(-16.5,12.85,22.2)) ;
#9983=CARTESIAN_POINT('Origin',(-16.5,12.2182755082439,18.0689260404997)) ;
#9984=CARTESIAN_POINT('',(-16.3,10.7319977197221,22.1880843115736)) ;
#9985=CARTESIAN_POINT('Origin',(-16.3,12.2182755082439,18.0689260404997)) ;
#9986=CARTESIAN_POINT('',(-16.5,10.8,22.)) ;
#9987=CARTESIAN_POINT('Ctrl Pts',(-16.3,10.7319962300621,22.188083771842)) ;
#9988=CARTESIAN_POINT('Ctrl Pts',(-16.3,10.7325345967251,22.1865948017166)) ;
#9989=CARTESIAN_POINT('Ctrl Pts',(-16.3000188015201,10.7330729440135,22.1851058840645)) ;
#9990=CARTESIAN_POINT('Ctrl Pts',(-16.3006567864184,10.7422054211292,22.1598480046429)) ;
#9991=CARTESIAN_POINT('Ctrl Pts',(-16.306044429893,10.7506834755747,22.1363998527687)) ;
#9992=CARTESIAN_POINT('Ctrl Pts',(-16.3261195505325,10.7667448574687,22.0919777741593)) ;
#9993=CARTESIAN_POINT('Ctrl Pts',(-16.3408899811084,10.7741400552678,22.0715241613828)) ;
#9994=CARTESIAN_POINT('Ctrl Pts',(-16.3779363523888,10.7865890441552,22.0370925871774)) ;
#9995=CARTESIAN_POINT('Ctrl Pts',(-16.3998581079217,10.7915238186497,22.0234438094466)) ;
#9996=CARTESIAN_POINT('Ctrl Pts',(-16.4480309426183,10.798258479926,22.0048167970752)) ;
#9997=CARTESIAN_POINT('Ctrl Pts',(-16.4738214623161,10.7999939814404,22.0000166464488)) ;
#9998=CARTESIAN_POINT('Ctrl Pts',(-16.4999096104036,10.7999999947913,22.0000000144066)) ;
#9999=CARTESIAN_POINT('Ctrl Pts',(-16.4999548051947,10.8,22.)) ;
#10000=CARTESIAN_POINT('Ctrl Pts',(-16.5,10.8,22.)) ;
#10001=CARTESIAN_POINT('Origin',(-16.5,12.2182755082439,18.0689260404997)) ;
#10002=CARTESIAN_POINT('Origin',(-16.5,7.48858533183141,21.0129348956712)) ;
#10003=CARTESIAN_POINT('',(-16.5,3.9,19.5)) ;
#10004=CARTESIAN_POINT('',(-16.5,7.5567150872414,20.8248967707396)) ;
#10005=CARTESIAN_POINT('',(-16.3,3.86223646644424,19.6990403792266)) ;
#10006=CARTESIAN_POINT('',(-16.3,7.48858533183141,21.0129348956712)) ;
#10007=CARTESIAN_POINT('Ctrl Pts',(-16.3,3.86223646644424,19.6990403792266)) ;
#10008=CARTESIAN_POINT('Ctrl Pts',(-16.3,3.86239942575251,19.6980436824249)) ;
#10009=CARTESIAN_POINT('Ctrl Pts',(-16.3000073893637,3.86256289052269,19.6970470816371)) ;
#10010=CARTESIAN_POINT('Ctrl Pts',(-16.300415494326,3.86708910313053,19.6695382704772)) ;
#10011=CARTESIAN_POINT('Ctrl Pts',(-16.3060387827755,3.87175164288346,19.6434145527853)) ;
#10012=CARTESIAN_POINT('Ctrl Pts',(-16.3269910238586,3.88069316641222,19.595511341096)) ;
#10013=CARTESIAN_POINT('Ctrl Pts',(-16.3418706315149,3.88489021711546,19.5740942364014)) ;
#10014=CARTESIAN_POINT('Ctrl Pts',(-16.3789985932666,3.8920605693635,19.5382677000811)) ;
#10015=CARTESIAN_POINT('Ctrl Pts',(-16.4008118680422,3.89497313876539,19.5241432650165)) ;
#10016=CARTESIAN_POINT('Ctrl Pts',(-16.4486601696573,3.89895928341784,19.5049329178167)) ;
#10017=CARTESIAN_POINT('Ctrl Pts',(-16.4742006804809,3.9,19.5)) ;
#10018=CARTESIAN_POINT('Ctrl Pts',(-16.5,3.9,19.5)) ;
#10019=CARTESIAN_POINT('Origin',(-16.5,3.86867726849999,19.973346585625)) ;
#10020=CARTESIAN_POINT('Origin',(-16.5,3.86867726849999,19.973346585625)) ;
#10021=CARTESIAN_POINT('Origin',(-16.3,3.86867726849999,19.973346585625)) ;
#10022=CARTESIAN_POINT('Origin',(-24.25,3.86867726849999,19.973346585625)) ;
#10023=CARTESIAN_POINT('',(-24.05,3.4,19.9)) ;
#10024=CARTESIAN_POINT('',(-24.25,3.4,19.9)) ;
#10025=CARTESIAN_POINT('',(-24.05,3.9,19.5)) ;
#10026=CARTESIAN_POINT('Origin',(-24.05,3.86867726849999,19.973346585625)) ;
#10027=CARTESIAN_POINT('',(-24.25,3.9,19.5)) ;
#10028=CARTESIAN_POINT('Origin',(-24.25,3.4,24.8)) ;
#10029=CARTESIAN_POINT('',(-24.05,3.4,24.8)) ;
#10030=CARTESIAN_POINT('',(-24.25,3.4,24.8)) ;
#10031=CARTESIAN_POINT('',(-24.05,3.4,5.91295268594296)) ;
#10032=CARTESIAN_POINT('Origin',(-24.25,3.73135783556136,24.8276015460276)) ;
#10033=CARTESIAN_POINT('',(-24.05,3.65,25.15)) ;
#10034=CARTESIAN_POINT('',(-24.25,3.65,25.15)) ;
#10035=CARTESIAN_POINT('Origin',(-24.05,3.73135783556136,24.8276015460276)) ;
#10036=CARTESIAN_POINT('Origin',(-24.25,8.9,27.05)) ;
#10037=CARTESIAN_POINT('',(-24.05,8.9,27.05)) ;
#10038=CARTESIAN_POINT('',(-24.25,8.9,27.05)) ;
#10039=CARTESIAN_POINT('',(-24.05,9.14517170941122,27.1387288091202)) ;
#10040=CARTESIAN_POINT('Origin',(-24.25,6.94557266623349,32.0941410006498)) ;
#10041=CARTESIAN_POINT('',(-24.05,10.85,28.35)) ;
#10042=CARTESIAN_POINT('',(-24.25,10.85,28.35)) ;
#10043=CARTESIAN_POINT('Origin',(-24.05,6.94557266623349,32.0941410006498)) ;
#10044=CARTESIAN_POINT('Origin',(-24.25,11.8,29.75)) ;
#10045=CARTESIAN_POINT('',(-24.05,11.8,29.75)) ;
#10046=CARTESIAN_POINT('',(-24.25,11.8,29.75)) ;
#10047=CARTESIAN_POINT('',(-24.05,3.78826756115411,17.9432364059113)) ;
#10048=CARTESIAN_POINT('Origin',(-24.25,17.5172318824408,27.2801860892852)) ;
#10049=CARTESIAN_POINT('',(-24.05,17.2,33.5)) ;
#10050=CARTESIAN_POINT('',(-24.25,17.2,33.5)) ;
#10051=CARTESIAN_POINT('Origin',(-24.05,17.5172318824408,27.2801860892852)) ;
#10052=CARTESIAN_POINT('Origin',(-24.25,17.2261159840305,33.8238840159695)) ;
#10053=CARTESIAN_POINT('',(-24.05,17.55,33.85)) ;
#10054=CARTESIAN_POINT('',(-24.25,17.55,33.85)) ;
#10055=CARTESIAN_POINT('Origin',(-24.05,17.2261159840305,33.8238840159695)) ;
#10056=CARTESIAN_POINT('Origin',(-24.25,17.55,37.8)) ;
#10057=CARTESIAN_POINT('',(-24.05,17.55,37.8)) ;
#10058=CARTESIAN_POINT('',(-24.25,17.55,37.8)) ;
#10059=CARTESIAN_POINT('',(-24.05,17.55,12.412952685943)) ;
#10060=CARTESIAN_POINT('Origin',(-24.25,18.75,37.7899579831933)) ;
#10061=CARTESIAN_POINT('',(-24.05,19.95,37.8)) ;
#10062=CARTESIAN_POINT('',(-24.25,19.95,37.8)) ;
#10063=CARTESIAN_POINT('Origin',(-24.05,18.75,37.7899579831933)) ;
#10064=CARTESIAN_POINT('Origin',(-24.25,19.95,34.)) ;
#10065=CARTESIAN_POINT('',(-24.05,19.95,34.)) ;
#10066=CARTESIAN_POINT('',(-24.25,19.95,34.)) ;
#10067=CARTESIAN_POINT('',(-24.05,19.95,10.512952685943)) ;
#10068=CARTESIAN_POINT('Origin',(-24.25,21.6437725346931,34.0916800205589)) ;
#10069=CARTESIAN_POINT('',(-24.05,20.75,32.65)) ;
#10070=CARTESIAN_POINT('',(-24.25,20.75,32.65)) ;
#10071=CARTESIAN_POINT('Origin',(-24.05,21.6437725346931,34.0916800205589)) ;
#10072=CARTESIAN_POINT('Origin',(-24.25,17.453364864871,27.1098816953352)) ;
#10073=CARTESIAN_POINT('',(-24.05,23.9,27.15)) ;
#10074=CARTESIAN_POINT('',(-24.25,23.9,27.15)) ;
#10075=CARTESIAN_POINT('Origin',(-24.05,17.453364864871,27.1098816953352)) ;
#10076=CARTESIAN_POINT('Origin',(-24.25,23.9,16.95)) ;
#10077=CARTESIAN_POINT('',(-24.05,23.9,16.95)) ;
#10078=CARTESIAN_POINT('',(-24.25,23.9,16.95)) ;
#10079=CARTESIAN_POINT('',(-24.05,23.9,1.98795268594296)) ;
#10080=CARTESIAN_POINT('Origin',(-24.25,33.4726637867458,16.9651420152427)) ;
#10081=CARTESIAN_POINT('',(-24.05,26.7,10.2)) ;
#10082=CARTESIAN_POINT('',(-24.25,26.7,10.2)) ;
#10083=CARTESIAN_POINT('Origin',(-24.05,33.4726637867458,16.9651420152427)) ;
#10084=CARTESIAN_POINT('Origin',(-16.3,23.9394766127413,-12.9740946281141)) ;
#10085=CARTESIAN_POINT('',(-16.3,19.6,36.797821691004)) ;
#10086=CARTESIAN_POINT('',(-16.3,19.6,37.802178308996)) ;
#10087=CARTESIAN_POINT('',(-16.3,19.6,12.412952685943)) ;
#10088=CARTESIAN_POINT('',(-16.3,17.9,36.797821691004)) ;
#10089=CARTESIAN_POINT('Origin',(-16.3,18.75,36.8151771653543)) ;
#10090=CARTESIAN_POINT('',(-16.3,17.9,37.8021783089959)) ;
#10091=CARTESIAN_POINT('',(-16.3,17.9,11.912952685943)) ;
#10092=CARTESIAN_POINT('Origin',(-16.3,18.75,37.7848228346457)) ;
#10093=CARTESIAN_POINT('',(-16.3,17.565,31.11)) ;
#10094=CARTESIAN_POINT('Origin',(-16.3,17.565,27.14)) ;
#10095=CARTESIAN_POINT('Origin',(-24.05,3.86867726849999,19.973346585625)) ;
#10096=CARTESIAN_POINT('',(-24.25,3.6,19.9176877660975)) ;
#10097=CARTESIAN_POINT('',(-24.25,3.86223646644423,19.6990403792266)) ;
#10098=CARTESIAN_POINT('Origin',(-24.25,3.86867726849999,19.973346585625)) ;
#10099=CARTESIAN_POINT('Ctrl Pts',(-24.25,3.86223646644423,19.6990403792266)) ;
#10100=CARTESIAN_POINT('Ctrl Pts',(-24.25,3.86239942575245,19.6980436824252)) ;
#10101=CARTESIAN_POINT('Ctrl Pts',(-24.2499926106363,3.86256289052268,19.6970470816371)) ;
#10102=CARTESIAN_POINT('Ctrl Pts',(-24.2495845056741,3.86708910312927,19.6695382704806)) ;
#10103=CARTESIAN_POINT('Ctrl Pts',(-24.2439612172248,3.87175164288334,19.643414552786)) ;
#10104=CARTESIAN_POINT('Ctrl Pts',(-24.2230089761414,3.88069316641219,19.595511341096)) ;
#10105=CARTESIAN_POINT('Ctrl Pts',(-24.2081293684851,3.88489021711545,19.5740942364014)) ;
#10106=CARTESIAN_POINT('Ctrl Pts',(-24.1710014067334,3.89206056936349,19.5382677000811)) ;
#10107=CARTESIAN_POINT('Ctrl Pts',(-24.1491881319578,3.89497313876537,19.5241432650165)) ;
#10108=CARTESIAN_POINT('Ctrl Pts',(-24.1013398303427,3.89895928341784,19.5049329178167)) ;
#10109=CARTESIAN_POINT('Ctrl Pts',(-24.0757993195191,3.89999999999997,19.5)) ;
#10110=CARTESIAN_POINT('Ctrl Pts',(-24.05,3.89999999999998,19.5)) ;
#10111=CARTESIAN_POINT('Ctrl Pts',(-24.25,3.6,19.9176877660975)) ;
#10112=CARTESIAN_POINT('Ctrl Pts',(-24.25,3.59869799800577,19.9175543222483)) ;
#10113=CARTESIAN_POINT('Ctrl Pts',(-24.2499872859315,3.59739597782284,19.9174213564527)) ;
#10114=CARTESIAN_POINT('Ctrl Pts',(-24.2494587398944,3.57033697971399,19.9146677791385)) ;
#10115=CARTESIAN_POINT('Ctrl Pts',(-24.2439832577742,3.54489668568231,19.9122633488296)) ;
#10116=CARTESIAN_POINT('Ctrl Pts',(-24.2235688176458,3.49728852286699,19.9079677236395)) ;
#10117=CARTESIAN_POINT('Ctrl Pts',(-24.2087545540871,3.4756013478467,19.9061195584593)) ;
#10118=CARTESIAN_POINT('Ctrl Pts',(-24.1716652613261,3.4391536116184,19.90309493138)) ;
#10119=CARTESIAN_POINT('Ctrl Pts',(-24.1497694510925,3.42472405685893,19.9019445727726)) ;
#10120=CARTESIAN_POINT('Ctrl Pts',(-24.1016856657977,3.40505796847904,19.9003903114039)) ;
#10121=CARTESIAN_POINT('Ctrl Pts',(-24.0759688441458,3.4,19.9)) ;
#10122=CARTESIAN_POINT('Ctrl Pts',(-24.05,3.4,19.9)) ;
#10123=CARTESIAN_POINT('Origin',(-24.05,7.48858533183141,21.0129348956712)) ;
#10124=CARTESIAN_POINT('',(-24.25,10.731997720549,22.1880843096407)) ;
#10125=CARTESIAN_POINT('',(-24.25,7.48858533183141,21.0129348956712)) ;
#10126=CARTESIAN_POINT('',(-24.05,10.8,22.)) ;
#10127=CARTESIAN_POINT('Ctrl Pts',(-24.25,10.7319962300761,22.1880837718459)) ;
#10128=CARTESIAN_POINT('Ctrl Pts',(-24.25,10.7325345967038,22.186594801818)) ;
#10129=CARTESIAN_POINT('Ctrl Pts',(-24.2499811984774,10.7330729441278,22.1851058839927)) ;
#10130=CARTESIAN_POINT('Ctrl Pts',(-24.2493432136556,10.7422054198757,22.1598480075178)) ;
#10131=CARTESIAN_POINT('Ctrl Pts',(-24.2439555708189,10.750683475002,22.136399854346)) ;
#10132=CARTESIAN_POINT('Ctrl Pts',(-24.2238804494726,10.7667448574682,22.0919777741686)) ;
#10133=CARTESIAN_POINT('Ctrl Pts',(-24.2091100188948,10.7741400552664,22.0715241613855)) ;
#10134=CARTESIAN_POINT('Ctrl Pts',(-24.172063647609,10.7865890441546,22.0370925871751)) ;
#10135=CARTESIAN_POINT('Ctrl Pts',(-24.1501418920773,10.7915238186451,22.0234438094444)) ;
#10136=CARTESIAN_POINT('Ctrl Pts',(-24.1019690573815,10.7982584799182,22.0048167970724)) ;
#10137=CARTESIAN_POINT('Ctrl Pts',(-24.0761785376837,10.7999939814428,22.0000166464497)) ;
#10138=CARTESIAN_POINT('Ctrl Pts',(-24.0500903895948,10.7999999947913,22.0000000144066)) ;
#10139=CARTESIAN_POINT('Ctrl Pts',(-24.050045194802,10.8,22.)) ;
#10140=CARTESIAN_POINT('Ctrl Pts',(-24.05,10.8,22.)) ;
#10141=CARTESIAN_POINT('',(-24.05,7.5567150872414,20.8248967707396)) ;
#10142=CARTESIAN_POINT('Origin',(-24.05,12.2182755082439,18.0689260404997)) ;
#10143=CARTESIAN_POINT('',(-24.25,12.9183976933795,22.3916931443706)) ;
#10144=CARTESIAN_POINT('Origin',(-24.25,12.2182755082439,18.0689260404997)) ;
#10145=CARTESIAN_POINT('',(-24.05,12.85,22.2)) ;
#10146=CARTESIAN_POINT('Ctrl Pts',(-24.25,12.9183976933795,22.3916931443706)) ;
#10147=CARTESIAN_POINT('Ctrl Pts',(-24.25,12.9181668378948,22.3910505718121)) ;
#10148=CARTESIAN_POINT('Ctrl Pts',(-24.2499966210206,12.9179359974498,22.3904079978316)) ;
#10149=CARTESIAN_POINT('Ctrl Pts',(-24.2497234095994,12.9086042548365,22.364430144348)) ;
#10150=CARTESIAN_POINT('Ctrl Pts',(-24.2442064359481,12.8996217972306,22.3393547558271)) ;
#10151=CARTESIAN_POINT('Ctrl Pts',(-24.223337166426,12.8830080878035,22.2928623998987)) ;
#10152=CARTESIAN_POINT('Ctrl Pts',(-24.2082563986562,12.8755130699976,22.271828861589)) ;
#10153=CARTESIAN_POINT('Ctrl Pts',(-24.1706426816821,12.8630621954662,22.2368282591497)) ;
#10154=CARTESIAN_POINT('Ctrl Pts',(-24.1486086719302,12.858181652241,22.2230759619812)) ;
#10155=CARTESIAN_POINT('Ctrl Pts',(-24.1007404646662,12.8516575377895,22.2046806927339)) ;
#10156=CARTESIAN_POINT('Ctrl Pts',(-24.0755026160457,12.85,22.2)) ;
#10157=CARTESIAN_POINT('Ctrl Pts',(-24.05,12.85,22.2)) ;
#10158=CARTESIAN_POINT('Origin',(-24.05,12.2182755082439,18.0689260404997)) ;
#10159=CARTESIAN_POINT('Origin',(-24.05,24.7469152941988,15.4731262457782)) ;
#10160=CARTESIAN_POINT('',(-24.25,15.63399980594,20.8033220974013)) ;
#10161=CARTESIAN_POINT('',(-24.25,24.7469152941988,15.4731262457782)) ;
#10162=CARTESIAN_POINT('',(-24.05,15.5,20.65)) ;
#10163=CARTESIAN_POINT('Ctrl Pts',(-24.25,15.63399980594,20.8033220974013)) ;
#10164=CARTESIAN_POINT('Ctrl Pts',(-24.25,15.6335509952832,20.8028060276234)) ;
#10165=CARTESIAN_POINT('Ctrl Pts',(-24.2499966124945,15.6331021746881,20.8022899714547)) ;
#10166=CARTESIAN_POINT('Ctrl Pts',(-24.249722940117,15.614972088751,20.7814449197118)) ;
#10167=CARTESIAN_POINT('Ctrl Pts',(-24.2442012683717,15.5974573764528,20.7613477431599)) ;
#10168=CARTESIAN_POINT('Ctrl Pts',(-24.2233158935857,15.5649632480559,20.7241280374561)) ;
#10169=CARTESIAN_POINT('Ctrl Pts',(-24.2082248717087,15.5502511678181,20.7073104617596)) ;
#10170=CARTESIAN_POINT('Ctrl Pts',(-24.1705925293635,15.5257656936601,20.6793548187585)) ;
#10171=CARTESIAN_POINT('Ctrl Pts',(-24.1485538369899,15.5161408054958,20.6683845338974)) ;
#10172=CARTESIAN_POINT('Ctrl Pts',(-24.1006977684759,15.5032739399685,20.653725811144)) ;
#10173=CARTESIAN_POINT('Ctrl Pts',(-24.0754813864138,15.5,20.65)) ;
#10174=CARTESIAN_POINT('Ctrl Pts',(-24.05,15.5,20.65)) ;
#10175=CARTESIAN_POINT('',(-24.05,24.6459386311912,15.3004887251523)) ;
#10176=CARTESIAN_POINT('Origin',(-24.05,12.5256959686759,18.3486581187154)) ;
#10177=CARTESIAN_POINT('',(-24.25,16.39481890426,19.1953078115317)) ;
#10178=CARTESIAN_POINT('Origin',(-24.25,12.5256959686759,18.3486581187154)) ;
#10179=CARTESIAN_POINT('',(-24.05,16.2,19.15)) ;
#10180=CARTESIAN_POINT('Ctrl Pts',(-24.25,16.39481890426,19.1953078115317)) ;
#10181=CARTESIAN_POINT('Ctrl Pts',(-24.25,16.3937985287439,19.195070324616)) ;
#10182=CARTESIAN_POINT('Ctrl Pts',(-24.2499917696977,16.3927781683397,19.1948328440442)) ;
#10183=CARTESIAN_POINT('Ctrl Pts',(-24.2495687833023,16.3665596763747,19.1887307763402)) ;
#10184=CARTESIAN_POINT('Ctrl Pts',(-24.2441462640923,16.3416754708443,19.1829410368979)) ;
#10185=CARTESIAN_POINT('Ctrl Pts',(-24.2238050373329,16.2951486910567,19.1721187037123)) ;
#10186=CARTESIAN_POINT('Ctrl Pts',(-24.2090186613912,16.2739730545514,19.1671947135444)) ;
#10187=CARTESIAN_POINT('Ctrl Pts',(-24.1719464410901,16.2383357459206,19.1589095136144)) ;
#10188=CARTESIAN_POINT('Ctrl Pts',(-24.150015697699,16.2242141206252,19.1556273129937)) ;
#10189=CARTESIAN_POINT('Ctrl Pts',(-24.1018323209062,16.2049543635143,19.1511512193477)) ;
#10190=CARTESIAN_POINT('Ctrl Pts',(-24.0760407121131,16.2,19.15)) ;
#10191=CARTESIAN_POINT('Ctrl Pts',(-24.05,16.2,19.15)) ;
#10192=CARTESIAN_POINT('Origin',(-24.05,12.5256959686759,18.3486581187154)) ;
#10193=CARTESIAN_POINT('Origin',(-24.05,17.75,12.412952685943)) ;
#10194=CARTESIAN_POINT('',(-24.25,17.75,37.799163194566)) ;
#10195=CARTESIAN_POINT('Ctrl Pts',(-24.05,17.55,37.8)) ;
#10196=CARTESIAN_POINT('Ctrl Pts',(-24.0632701694844,17.55,37.7999646531197)) ;
#10197=CARTESIAN_POINT('Ctrl Pts',(-24.0765399924102,17.5513250740506,37.7999293062395)) ;
#10198=CARTESIAN_POINT('Ctrl Pts',(-24.0895481340208,17.5539491262568,37.7998939593592)) ;
#10199=CARTESIAN_POINT('Ctrl Pts',(-24.1025532968563,17.5565725775731,37.7998586205732)) ;
#10200=CARTESIAN_POINT('Ctrl Pts',(-24.1152962197139,17.5604942733101,37.7998232817871)) ;
#10201=CARTESIAN_POINT('Ctrl Pts',(-24.1275260588055,17.5656370150868,37.799787943001)) ;
#10202=CARTESIAN_POINT('Ctrl Pts',(-24.1397534773073,17.5707787389869,37.7997526112094)) ;
#10203=CARTESIAN_POINT('Ctrl Pts',(-24.1514673780366,17.5771407558669,37.7997172794177)) ;
#10204=CARTESIAN_POINT('Ctrl Pts',(-24.1624372641837,17.5845978790254,37.7996819476261)) ;
#10205=CARTESIAN_POINT('Ctrl Pts',(-24.1734053194263,17.5920537575693,37.7996466217314)) ;
#10206=CARTESIAN_POINT('Ctrl Pts',(-24.1836290375724,17.6006039870742,37.7996112958368)) ;
#10207=CARTESIAN_POINT('Ctrl Pts',(-24.1929073111899,17.6100803787581,37.7995759699421)) ;
#10208=CARTESIAN_POINT('Ctrl Pts',(-24.2021908572985,17.6195621555162,37.7995406239731)) ;
#10209=CARTESIAN_POINT('Ctrl Pts',(-24.2105273961139,17.6299706560222,37.7995052780041)) ;
#10210=CARTESIAN_POINT('Ctrl Pts',(-24.2177527569689,17.6411009066643,37.799469932035)) ;
#10211=CARTESIAN_POINT('Ctrl Pts',(-24.2249750808544,17.6522264790305,37.7994346009226)) ;
#10212=CARTESIAN_POINT('Ctrl Pts',(-24.2310867869367,17.6640726125166,37.7993992698103)) ;
#10213=CARTESIAN_POINT('Ctrl Pts',(-24.2359676185276,17.6764062172518,37.7993639386979)) ;
#10214=CARTESIAN_POINT('Ctrl Pts',(-24.2408502551657,17.6887443832466,37.7993285945192)) ;
#10215=CARTESIAN_POINT('Ctrl Pts',(-24.2445008489509,17.7015697384064,37.7992932503405)) ;
#10216=CARTESIAN_POINT('Ctrl Pts',(-24.2468475163264,17.7146297396653,37.7992579061619)) ;
#10217=CARTESIAN_POINT('Ctrl Pts',(-24.2489436334282,17.7262953435236,37.7992263356299)) ;
#10218=CARTESIAN_POINT('Ctrl Pts',(-24.25,17.7381475732323,37.799194765098)) ;
#10219=CARTESIAN_POINT('Ctrl Pts',(-24.25,17.75,37.799163194566)) ;
#10220=CARTESIAN_POINT('',(-24.25,17.75,33.8570883563437)) ;
#10221=CARTESIAN_POINT('',(-24.25,17.75,12.412952685943)) ;
#10222=CARTESIAN_POINT('Ctrl Pts',(-24.25,17.75,33.8570883563437)) ;
#10223=CARTESIAN_POINT('Ctrl Pts',(-24.25,17.7483048927981,33.8570346913132)) ;
#10224=CARTESIAN_POINT('Ctrl Pts',(-24.2499784495869,17.7466098579761,33.8569808984569)) ;
#10225=CARTESIAN_POINT('Ctrl Pts',(-24.2492934706748,17.7196757862012,33.8561240343194)) ;
#10226=CARTESIAN_POINT('Ctrl Pts',(-24.2438780635363,17.6947845328972,33.8553018126003)) ;
#10227=CARTESIAN_POINT('Ctrl Pts',(-24.2237614818921,17.6476026569698,33.8536820465369)) ;
#10228=CARTESIAN_POINT('Ctrl Pts',(-24.2089645660017,17.6258680589014,33.8529014445044)) ;
#10229=CARTESIAN_POINT('Ctrl Pts',(-24.1718827931726,17.5893078527847,33.8515452810162)) ;
#10230=CARTESIAN_POINT('Ctrl Pts',(-24.1499574522595,17.5748252688856,33.8509836241205)) ;
#10231=CARTESIAN_POINT('Ctrl Pts',(-24.1017958701297,17.555078893135,33.8502065060916)) ;
#10232=CARTESIAN_POINT('Ctrl Pts',(-24.0760230373047,17.55,33.85)) ;
#10233=CARTESIAN_POINT('Ctrl Pts',(-24.05,17.55,33.85)) ;
#10234=CARTESIAN_POINT('Origin',(-24.05,29.7633733578399,-15.291248496029)) ;
#10235=CARTESIAN_POINT('',(-24.05,35.4,-9.7)) ;
#10236=CARTESIAN_POINT('',(-24.25,35.541707130624,-9.55886443234855)) ;
#10237=CARTESIAN_POINT('Ctrl Pts',(-24.05,35.4,-9.7)) ;
#10238=CARTESIAN_POINT('Ctrl Pts',(-24.0632701694643,35.3999882729118,-9.69998817773565)) ;
#10239=CARTESIAN_POINT('Ctrl Pts',(-24.0765399923701,35.4009172937257,-9.6990431810638)) ;
#10240=CARTESIAN_POINT('Ctrl Pts',(-24.0895481339619,35.4027685180476,-9.69718337031635)) ;
#10241=CARTESIAN_POINT('Ctrl Pts',(-24.1025532967779,35.4046193184517,-9.6953239854529)) ;
#10242=CARTESIAN_POINT('Ctrl Pts',(-24.1152962196173,35.4073918013753,-9.69255030317433)) ;
#10243=CARTESIAN_POINT('Ctrl Pts',(-24.1275260586929,35.4110311429201,-9.68891667355651)) ;
#10244=CARTESIAN_POINT('Ctrl Pts',(-24.139753477178,35.4146697641483,-9.68528376312474)) ;
#10245=CARTESIAN_POINT('Ctrl Pts',(-24.1514673778929,35.4191747093011,-9.68079143563539)) ;
#10246=CARTESIAN_POINT('Ctrl Pts',(-24.1624372640292,35.4244570869814,-9.67552783886286)) ;
#10247=CARTESIAN_POINT('Ctrl Pts',(-24.1734053192599,35.4297385830177,-9.67026512059973)) ;
#10248=CARTESIAN_POINT('Ctrl Pts',(-24.1836290373979,35.4357969752947,-9.66423166493807)) ;
#10249=CARTESIAN_POINT('Ctrl Pts',(-24.1929073110115,35.4425128458928,-9.65754590678402)) ;
#10250=CARTESIAN_POINT('Ctrl Pts',(-24.2021908571152,35.4492325328647,-9.65085634936783)) ;
#10251=CARTESIAN_POINT('Ctrl Pts',(-24.2105273959302,35.4566100967359,-9.64351409386539)) ;
#10252=CARTESIAN_POINT('Ctrl Pts',(-24.2177527567903,35.4645000078171,-9.63566348462498)) ;
#10253=CARTESIAN_POINT('Ctrl Pts',(-24.2249750806803,35.4723866026039,-9.62781617515956)) ;
#10254=CARTESIAN_POINT('Ctrl Pts',(-24.2310867867725,35.4807847004745,-9.61946134933943)) ;
#10255=CARTESIAN_POINT('Ctrl Pts',(-24.235967618379,35.4895288148778,-9.61076315675825)) ;
#10256=CARTESIAN_POINT('Ctrl Pts',(-24.2408502550324,35.4982761630614,-9.6020617473797)) ;
#10257=CARTESIAN_POINT('Ctrl Pts',(-24.2445008488388,35.5073693274479,-9.5930171698336)) ;
#10258=CARTESIAN_POINT('Ctrl Pts',(-24.2468475162411,35.5166290153408,-9.58380727835446)) ;
#10259=CARTESIAN_POINT('Ctrl Pts',(-24.2489436333995,35.52490005991,-9.57558071350875)) ;
#10260=CARTESIAN_POINT('Ctrl Pts',(-24.25,35.5333035489127,-9.56722266607385)) ;
#10261=CARTESIAN_POINT('Ctrl Pts',(-24.25,35.541707130624,-9.55886443234855)) ;
#10262=CARTESIAN_POINT('',(-24.25,37.8999308547965,-15.5052586405422)) ;
#10263=CARTESIAN_POINT('Origin',(-24.25,29.7633733578399,-15.291248496029)) ;
#10264=CARTESIAN_POINT('',(-24.05,37.7,-15.5)) ;
#10265=CARTESIAN_POINT('Origin',(-24.05,37.8999308547965,-15.5052586405422)) ;
#10266=CARTESIAN_POINT('Origin',(-24.05,29.7633733578399,-15.291248496029)) ;
#10267=CARTESIAN_POINT('Origin',(-24.05,37.9279179147939,-14.4204278690655)) ;
#10268=CARTESIAN_POINT('',(-24.05,36.65,-56.2)) ;
#10269=CARTESIAN_POINT('',(-24.05,37.7279844379825,-14.415269880106)) ;
#10270=CARTESIAN_POINT('',(-24.25,36.8459456848986,-56.3597323992937)) ;
#10271=CARTESIAN_POINT('',(-24.25,37.9279179147939,-14.4204278690655)) ;
#10272=CARTESIAN_POINT('Ctrl Pts',(-24.25,36.8459456848986,-56.3597323992937)) ;
#10273=CARTESIAN_POINT('Ctrl Pts',(-24.25,36.8452932432196,-56.3591906677191)) ;
#10274=CARTESIAN_POINT('Ctrl Pts',(-24.2499966713728,36.8446407490717,-56.3586489949844)) ;
#10275=CARTESIAN_POINT('Ctrl Pts',(-24.2498073839985,36.826091678425,-56.3432532583288)) ;
#10276=CARTESIAN_POINT('Ctrl Pts',(-24.2471193144542,36.8081301664191,-56.3284236042304)) ;
#10277=CARTESIAN_POINT('Ctrl Pts',(-24.2367641356701,36.7736693811156,-56.3001110660321)) ;
#10278=CARTESIAN_POINT('Ctrl Pts',(-24.2292318720098,36.7570768798035,-56.2865472202178)) ;
#10279=CARTESIAN_POINT('Ctrl Pts',(-24.2064522017498,36.7216811428078,-56.2577328860845)) ;
#10280=CARTESIAN_POINT('Ctrl Pts',(-24.1896672437335,36.7034378018957,-56.2429732328781)) ;
#10281=CARTESIAN_POINT('Ctrl Pts',(-24.1519096063163,36.6760935350204,-56.220928962173)) ;
#10282=CARTESIAN_POINT('Ctrl Pts',(-24.132484884718,36.6660883821569,-56.2128959810192)) ;
#10283=CARTESIAN_POINT('Ctrl Pts',(-24.0915642364822,36.653234532305,-56.2025876834372)) ;
#10284=CARTESIAN_POINT('Ctrl Pts',(-24.0709835762204,36.65,-56.2)) ;
#10285=CARTESIAN_POINT('Ctrl Pts',(-24.05,36.65,-56.2)) ;
#10286=CARTESIAN_POINT('Origin',(-24.05,18.75,37.7899579831933)) ;
#10287=CARTESIAN_POINT('',(-24.25,19.7499996500575,37.7991631591148)) ;
#10288=CARTESIAN_POINT('Ctrl Pts',(-24.05,19.95,37.8)) ;
#10289=CARTESIAN_POINT('Ctrl Pts',(-24.0632701637967,19.9499996450624,37.8000424142976)) ;
#10290=CARTESIAN_POINT('Ctrl Pts',(-24.0765399810356,19.94867426136,37.8000737393719)) ;
#10291=CARTESIAN_POINT('Ctrl Pts',(-24.0895481172947,19.9460499473545,37.8000937776279)) ;
#10292=CARTESIAN_POINT('Ctrl Pts',(-24.1025532746016,19.9434262343348,37.8001138112951)) ;
#10293=CARTESIAN_POINT('Ctrl Pts',(-24.1152961922746,19.9395043247711,37.8001225626839)) ;
#10294=CARTESIAN_POINT('Ctrl Pts',(-24.1275260268481,19.9343614175846,37.8001202894756)) ;
#10295=CARTESIAN_POINT('Ctrl Pts',(-24.1397534405889,19.92921952841,37.8001180167172)) ;
#10296=CARTESIAN_POINT('Ctrl Pts',(-24.1514673372456,19.9228573947066,37.8001047243444)) ;
#10297=CARTESIAN_POINT('Ctrl Pts',(-24.1624372203003,19.915400201571,37.8000811250022)) ;
#10298=CARTESIAN_POINT('Ctrl Pts',(-24.1734052721897,19.9079442532392,37.8000575295993)) ;
#10299=CARTESIAN_POINT('Ctrl Pts',(-24.1836289879996,19.899394000828,37.8000236325339)) ;
#10300=CARTESIAN_POINT('Ctrl Pts',(-24.1929072605376,19.8899176293381,37.7999805824503)) ;
#10301=CARTESIAN_POINT('Ctrl Pts',(-24.2021908052356,19.8804358731232,37.7999375079045)) ;
#10302=CARTESIAN_POINT('Ctrl Pts',(-24.2105273439674,19.8700274363687,37.7998852729588)) ;
#10303=CARTESIAN_POINT('Ctrl Pts',(-24.2177527062381,19.8588972867723,37.7998254284371)) ;
#10304=CARTESIAN_POINT('Ctrl Pts',(-24.2249750314017,19.8477718156204,37.7997656090704)) ;
#10305=CARTESIAN_POINT('Ctrl Pts',(-24.231086740303,19.8359258206247,37.7996981907095)) ;
#10306=CARTESIAN_POINT('Ctrl Pts',(-24.2359675763273,19.8235923837952,37.7996250677075)) ;
#10307=CARTESIAN_POINT('Ctrl Pts',(-24.2408502173167,19.8112543859802,37.7995519176641)) ;
#10308=CARTESIAN_POINT('Ctrl Pts',(-24.2445008171118,19.7984292284339,37.7994730638621)) ;
#10309=CARTESIAN_POINT('Ctrl Pts',(-24.2468474921171,19.7853694446507,37.7993906788029)) ;
#10310=CARTESIAN_POINT('Ctrl Pts',(-24.2489436252733,19.7737039836308,37.7993170895528)) ;
#10311=CARTESIAN_POINT('Ctrl Pts',(-24.25,19.7618519109258,37.7992406894262)) ;
#10312=CARTESIAN_POINT('Ctrl Pts',(-24.25,19.7499996500575,37.7991631591148)) ;
#10313=CARTESIAN_POINT('Origin',(-24.25,18.75,37.7899579831933)) ;
#10314=CARTESIAN_POINT('Origin',(-24.05,37.7318176617063,-60.502128268216)) ;
#10315=CARTESIAN_POINT('',(-24.25,41.9506268879595,-60.8840463309467)) ;
#10316=CARTESIAN_POINT('Origin',(-24.25,37.7318176617063,-60.502128268216)) ;
#10317=CARTESIAN_POINT('',(-24.05,42.15,-60.9)) ;
#10318=CARTESIAN_POINT('Ctrl Pts',(-24.25,41.9506268879594,-60.8840463309467)) ;
#10319=CARTESIAN_POINT('Ctrl Pts',(-24.25,41.9517471911499,-60.8841361107773)) ;
#10320=CARTESIAN_POINT('Ctrl Pts',(-24.2499905274602,41.9528674746358,-60.884225886703)) ;
#10321=CARTESIAN_POINT('Ctrl Pts',(-24.2495367852489,41.9796968068967,-60.8863758483662)) ;
#10322=CARTESIAN_POINT('Ctrl Pts',(-24.2441168334782,42.0050812395976,-60.8884087660416)) ;
#10323=CARTESIAN_POINT('Ctrl Pts',(-24.2238077082346,42.0526243758534,-60.8922143172946)) ;
#10324=CARTESIAN_POINT('Ctrl Pts',(-24.2090218955104,42.074295218724,-60.893947902738)) ;
#10325=CARTESIAN_POINT('Ctrl Pts',(-24.1719501690967,42.1107665799089,-60.8968644715332)) ;
#10326=CARTESIAN_POINT('Ctrl Pts',(-24.1500190632069,42.1252187814051,-60.8980196294303)) ;
#10327=CARTESIAN_POINT('Ctrl Pts',(-24.1018344050974,42.1449296139692,-60.8995949062453)) ;
#10328=CARTESIAN_POINT('Ctrl Pts',(-24.0760417263098,42.15,-60.8999999999999)) ;
#10329=CARTESIAN_POINT('Ctrl Pts',(-24.05,42.1500000000001,-60.8999999999991)) ;
#10330=CARTESIAN_POINT('Origin',(-24.05,37.7318176617063,-60.502128268216)) ;
#10331=CARTESIAN_POINT('Origin',(-24.05,43.5701155187154,-37.6713759567788)) ;
#10332=CARTESIAN_POINT('',(-24.25,42.1003608664925,-58.7378593416195)) ;
#10333=CARTESIAN_POINT('',(-24.25,43.5701155187154,-37.6713759567788)) ;
#10334=CARTESIAN_POINT('',(-24.05,42.3,-58.75)) ;
#10335=CARTESIAN_POINT('Origin',(-24.05,42.1003608738345,-58.7378592000713)) ;
#10336=CARTESIAN_POINT('',(-24.05,43.7696305388826,-37.6852956093486)) ;
#10337=CARTESIAN_POINT('Origin',(-24.05,33.4726637867458,16.9651420152427)) ;
#10338=CARTESIAN_POINT('',(-24.25,23.7000000012803,16.9498418202582)) ;
#10339=CARTESIAN_POINT('Ctrl Pts',(-24.25,23.7000000012803,16.9498418202582)) ;
#10340=CARTESIAN_POINT('Ctrl Pts',(-24.25,23.7132701649591,16.9498559146256)) ;
#10341=CARTESIAN_POINT('Ctrl Pts',(-24.24867492595,23.7265399820437,16.9498700358474)) ;
#10342=CARTESIAN_POINT('Ctrl Pts',(-24.2460508737449,23.7395481180995,16.9498837737012)) ;
#10343=CARTESIAN_POINT('Ctrl Pts',(-24.2434274224297,23.7525532753816,16.9498975084091)) ;
#10344=CARTESIAN_POINT('Ctrl Pts',(-24.2395057266942,23.765296192973,16.9499108588538)) ;
#10345=CARTESIAN_POINT('Ctrl Pts',(-24.2343629849196,23.7775260273978,16.9499234291553)) ;
#10346=CARTESIAN_POINT('Ctrl Pts',(-24.2292212610216,23.7897534412339,16.9499359969688)) ;
#10347=CARTESIAN_POINT('Ctrl Pts',(-24.222859244144,23.8014673378977,16.949947783934)) ;
#10348=CARTESIAN_POINT('Ctrl Pts',(-24.2154021209883,23.8124372208699,16.9499584241338)) ;
#10349=CARTESIAN_POINT('Ctrl Pts',(-24.2079462424471,23.8234052729382,16.9499690625578)) ;
#10350=CARTESIAN_POINT('Ctrl Pts',(-24.1993960129453,23.8336289888011,16.9499785536818)) ;
#10351=CARTESIAN_POINT('Ctrl Pts',(-24.1899196212647,23.8429072612832,16.9499865760112)) ;
#10352=CARTESIAN_POINT('Ctrl Pts',(-24.1804378445097,23.8521908062561,16.9499946028994)) ;
#10353=CARTESIAN_POINT('Ctrl Pts',(-24.1700293440071,23.8605273450856,16.9500011585298)) ;
#10354=CARTESIAN_POINT('Ctrl Pts',(-24.1588990933682,23.8677527073182,16.9500059780284)) ;
#10355=CARTESIAN_POINT('Ctrl Pts',(-24.1477735210053,23.8749750325807,16.9500107955012)) ;
#10356=CARTESIAN_POINT('Ctrl Pts',(-24.1359273875225,23.8810867414029,16.9500138776823)) ;
#10357=CARTESIAN_POINT('Ctrl Pts',(-24.1235937827905,23.8859675772572,16.9500150277399)) ;
#10358=CARTESIAN_POINT('Ctrl Pts',(-24.1112556167988,23.8908502181604,16.9500161782227)) ;
#10359=CARTESIAN_POINT('Ctrl Pts',(-24.0984302616419,23.8945008177358,16.9500153947128)) ;
#10360=CARTESIAN_POINT('Ctrl Pts',(-24.0853702603857,23.8968474925285,16.9500125559086)) ;
#10361=CARTESIAN_POINT('Ctrl Pts',(-24.0737046565109,23.898943616259,16.9500100201995)) ;
#10362=CARTESIAN_POINT('Ctrl Pts',(-24.061852426785,23.8999999907535,16.9500058455726)) ;
#10363=CARTESIAN_POINT('Ctrl Pts',(-24.05,23.9,16.95)) ;
#10364=CARTESIAN_POINT('',(-24.25,26.5585000901577,10.0586572410252)) ;
#10365=CARTESIAN_POINT('Origin',(-24.05,26.5585000901577,10.0586572410252)) ;
#10366=CARTESIAN_POINT('Origin',(-24.25,33.4726637867458,16.9651420152427)) ;
#10367=CARTESIAN_POINT('Origin',(-24.05,37.4869714539765,-0.869814166451149)) ;
#10368=CARTESIAN_POINT('',(-24.05,38.35,-1.45)) ;
#10369=CARTESIAN_POINT('',(-24.25,38.2088062765873,-1.59164898906192)) ;
#10370=CARTESIAN_POINT('Ctrl Pts',(-24.05,38.35,-1.45)) ;
#10371=CARTESIAN_POINT('Ctrl Pts',(-24.0632701694844,38.35000961527,-1.45000961527001)) ;
#10372=CARTESIAN_POINT('Ctrl Pts',(-24.0765399924102,38.3490822616933,-1.45095619938675)) ;
#10373=CARTESIAN_POINT('Ctrl Pts',(-24.0895481340208,38.3472363918541,-1.45282129976597)) ;
#10374=CARTESIAN_POINT('Ctrl Pts',(-24.1025532968563,38.3453909447064,-1.45468597305001)) ;
#10375=CARTESIAN_POINT('Ctrl Pts',(-24.1152962197139,38.3426275001252,-1.4574686437676)) ;
#10376=CARTESIAN_POINT('Ctrl Pts',(-24.1275260588055,38.3390006456092,-1.46111472441998)) ;
#10377=CARTESIAN_POINT('Ctrl Pts',(-24.1397534773073,38.335374508938,-1.4647600834222)) ;
#10378=CARTESIAN_POINT('Ctrl Pts',(-24.1514673780366,38.3308854948256,-1.46926831986561)) ;
#10379=CARTESIAN_POINT('Ctrl Pts',(-24.1624372641837,38.3256221236376,-1.47455091338466)) ;
#10380=CARTESIAN_POINT('Ctrl Pts',(-24.1734053194263,38.3203596309209,-1.47983262522414)) ;
#10381=CARTESIAN_POINT('Ctrl Pts',(-24.1836290375724,38.3143233152186,-1.48588816004911)) ;
#10382=CARTESIAN_POINT('Ctrl Pts',(-24.1929073111898,38.3076321039592,-1.49259859043134)) ;
#10383=CARTESIAN_POINT('Ctrl Pts',(-24.2021908572985,38.3009370903379,-1.49931283409685)) ;
#10384=CARTESIAN_POINT('Ctrl Pts',(-24.2105273961138,38.2935867840703,-1.50668237040873)) ;
#10385=CARTESIAN_POINT('Ctrl Pts',(-24.2177527569689,38.2857261233871,-1.51456226113624)) ;
#10386=CARTESIAN_POINT('Ctrl Pts',(-24.2249750808544,38.2778687667031,-1.52243883978168)) ;
#10387=CARTESIAN_POINT('Ctrl Pts',(-24.2310867869367,38.269501896365,-1.53082493208131)) ;
#10388=CARTESIAN_POINT('Ctrl Pts',(-24.2359676185276,38.260790331801,-1.53955571860678)) ;
#10389=CARTESIAN_POINT('Ctrl Pts',(-24.2408502551657,38.2520755454938,-1.54828973398417)) ;
#10390=CARTESIAN_POINT('Ctrl Pts',(-24.2445008489509,38.2430162644243,-1.55736824412392)) ;
#10391=CARTESIAN_POINT('Ctrl Pts',(-24.2468475163264,38.2337910635069,-1.5666126741115)) ;
#10392=CARTESIAN_POINT('Ctrl Pts',(-24.2489436334282,38.2255508239172,-1.5748700897115)) ;
#10393=CARTESIAN_POINT('Ctrl Pts',(-24.25,38.2171786199231,-1.58325946971581)) ;
#10394=CARTESIAN_POINT('Ctrl Pts',(-24.25,38.2088062765873,-1.59164898906192)) ;
#10395=CARTESIAN_POINT('',(-24.25,37.4869714539765,-0.869814166451149)) ;
#10396=CARTESIAN_POINT('',(-24.05,37.6283928102138,-0.72839281021384)) ;
#10397=CARTESIAN_POINT('Origin',(-24.05,23.7,1.98795268594296)) ;
#10398=CARTESIAN_POINT('',(-24.25,23.6999999690425,27.1493776857403)) ;
#10399=CARTESIAN_POINT('',(-24.25,23.7,1.98795268594296)) ;
#10400=CARTESIAN_POINT('Ctrl Pts',(-24.25,23.7000000155168,27.1493727892866)) ;
#10401=CARTESIAN_POINT('Ctrl Pts',(-24.2499999998777,23.7015760333225,27.1493777710123)) ;
#10402=CARTESIAN_POINT('Ctrl Pts',(-24.2499813712591,23.703151980566,27.1493827515679)) ;
#10403=CARTESIAN_POINT('Ctrl Pts',(-24.2493452398792,23.7300560876817,27.1494677621689)) ;
#10404=CARTESIAN_POINT('Ctrl Pts',(-24.2439389270727,23.7550416809086,27.1495464596794)) ;
#10405=CARTESIAN_POINT('Ctrl Pts',(-24.2238108181396,23.802313411751,27.1496949552354)) ;
#10406=CARTESIAN_POINT('Ctrl Pts',(-24.2090255878345,23.824052809064,27.1497630282056)) ;
#10407=CARTESIAN_POINT('Ctrl Pts',(-24.1719543545186,23.8606404855449,27.1498773846942)) ;
#10408=CARTESIAN_POINT('Ctrl Pts',(-24.15002280892,23.8751390022258,27.1499225811516)) ;
#10409=CARTESIAN_POINT('Ctrl Pts',(-24.1018367027478,23.8949132761296,27.1499841811619)) ;
#10410=CARTESIAN_POINT('Ctrl Pts',(-24.0760428468437,23.9,27.1499999999993)) ;
#10411=CARTESIAN_POINT('Ctrl Pts',(-24.05,23.9,27.1499999999993)) ;
#10412=CARTESIAN_POINT('Origin',(-24.05,23.7122919887408,-16.1822567109578)) ;
#10413=CARTESIAN_POINT('',(-24.05,44.45,-17.3)) ;
#10414=CARTESIAN_POINT('',(-24.25,44.2502789868947,-17.2894378848858)) ;
#10415=CARTESIAN_POINT('Ctrl Pts',(-24.05,44.45,-17.3)) ;
#10416=CARTESIAN_POINT('Ctrl Pts',(-24.0632701694836,44.4499995354581,-17.3000086187351)) ;
#10417=CARTESIAN_POINT('Ctrl Pts',(-24.0765399924086,44.4486759174207,-17.2999459207093)) ;
#10418=CARTESIAN_POINT('Ctrl Pts',(-24.0895481340185,44.4460552042224,-17.2998133055442)) ;
#10419=CARTESIAN_POINT('Ctrl Pts',(-24.1025532968532,44.4434350911495,-17.299680720747)) ;
#10420=CARTESIAN_POINT('Ctrl Pts',(-24.1152962197101,44.4395186155883,-17.2994782582822)) ;
#10421=CARTESIAN_POINT('Ctrl Pts',(-24.127526058801,44.4343828642744,-17.2992100684806)) ;
#10422=CARTESIAN_POINT('Ctrl Pts',(-24.1397534773022,44.4292481294536,-17.2989419317604)) ;
#10423=CARTESIAN_POINT('Ctrl Pts',(-24.1514673780309,44.4228948708492,-17.2986081082184)) ;
#10424=CARTESIAN_POINT('Ctrl Pts',(-24.1624372641776,44.4154480939293,-17.2982153315896)) ;
#10425=CARTESIAN_POINT('Ctrl Pts',(-24.1734053194197,44.4080025598972,-17.2978226205164)) ;
#10426=CARTESIAN_POINT('Ctrl Pts',(-24.1836290375656,44.399464261773,-17.2973709969963)) ;
#10427=CARTESIAN_POINT('Ctrl Pts',(-24.1929073111829,44.39000114473,-17.2968695100719)) ;
#10428=CARTESIAN_POINT('Ctrl Pts',(-24.2021908572913,44.3805326501562,-17.2963677381714)) ;
#10429=CARTESIAN_POINT('Ctrl Pts',(-24.2105273961066,44.3701387759104,-17.2958160726108)) ;
#10430=CARTESIAN_POINT('Ctrl Pts',(-24.2177527569619,44.3590241986199,-17.2952255433351)) ;
#10431=CARTESIAN_POINT('Ctrl Pts',(-24.2249750808476,44.3479142930177,-17.2946352622711)) ;
#10432=CARTESIAN_POINT('Ctrl Pts',(-24.2310867869303,44.3360848716631,-17.2940061814933)) ;
#10433=CARTESIAN_POINT('Ctrl Pts',(-24.2359676185217,44.3237686866229,-17.2933508454617)) ;
#10434=CARTESIAN_POINT('Ctrl Pts',(-24.2408502551605,44.3114479467653,-17.2926952670713)) ;
#10435=CARTESIAN_POINT('Ctrl Pts',(-24.2445008489465,44.298640724898,-17.2920134485918)) ;
#10436=CARTESIAN_POINT('Ctrl Pts',(-24.246847516323,44.2855991980142,-17.2913189828271)) ;
#10437=CARTESIAN_POINT('Ctrl Pts',(-24.2489436334271,44.2739500960415,-17.2906986641649)) ;
#10438=CARTESIAN_POINT('Ctrl Pts',(-24.25,44.2621146394998,-17.2900682864539)) ;
#10439=CARTESIAN_POINT('Ctrl Pts',(-24.25,44.2502789868947,-17.2894378848858)) ;
#10440=CARTESIAN_POINT('Origin',(-24.25,23.7122919887408,-16.1822567109578)) ;
#10441=CARTESIAN_POINT('Origin',(-24.05,23.7122919887408,-16.1822567109578)) ;
#10442=CARTESIAN_POINT('Origin',(-24.05,17.453364864871,27.1098816953352)) ;
#10443=CARTESIAN_POINT('',(-24.25,20.6462198057264,32.4790238413936)) ;
#10444=CARTESIAN_POINT('Origin',(-24.25,17.453364864871,27.1098816953352)) ;
#10445=CARTESIAN_POINT('Ctrl Pts',(-24.25,20.6462198057264,32.4790238413936)) ;
#10446=CARTESIAN_POINT('Ctrl Pts',(-24.25,20.6467552570576,32.4799066099211)) ;
#10447=CARTESIAN_POINT('Ctrl Pts',(-24.2499920056975,20.6472907045759,32.4807893626782)) ;
#10448=CARTESIAN_POINT('Ctrl Pts',(-24.2495751592316,20.6612498771786,32.5038025845034)) ;
#10449=CARTESIAN_POINT('Ctrl Pts',(-24.2441531700626,20.6745092215521,32.5256560187645)) ;
#10450=CARTESIAN_POINT('Ctrl Pts',(-24.2238084309022,20.6992979967966,32.5665017098134)) ;
#10451=CARTESIAN_POINT('Ctrl Pts',(-24.2090227178855,20.71057946702,32.5850854157313)) ;
#10452=CARTESIAN_POINT('Ctrl Pts',(-24.1719510657226,20.7295683297316,32.6163598545375)) ;
#10453=CARTESIAN_POINT('Ctrl Pts',(-24.150019848274,20.7370942674122,32.6287518975251)) ;
#10454=CARTESIAN_POINT('Ctrl Pts',(-24.1018348748854,20.7473591548606,32.6456526691067)) ;
#10455=CARTESIAN_POINT('Ctrl Pts',(-24.0760419567382,20.75,32.65)) ;
#10456=CARTESIAN_POINT('Ctrl Pts',(-24.05,20.75,32.65)) ;
#10457=CARTESIAN_POINT('Origin',(-24.05,43.2596418025572,-36.388001295162)) ;
#10458=CARTESIAN_POINT('',(-24.25,43.2596418025572,-36.388001295162)) ;
#10459=CARTESIAN_POINT('',(-24.05,43.4593732974275,-36.3983613123869)) ;
#10460=CARTESIAN_POINT('Origin',(-24.05,21.6437725346931,34.0916800205589)) ;
#10461=CARTESIAN_POINT('',(-24.25,19.75,33.9947419676037)) ;
#10462=CARTESIAN_POINT('Origin',(-24.25,21.6437725346931,34.0916800205589)) ;
#10463=CARTESIAN_POINT('Ctrl Pts',(-24.25,19.75,33.9947419676037)) ;
#10464=CARTESIAN_POINT('Ctrl Pts',(-24.25,19.7510782785915,33.9947695469051)) ;
#10465=CARTESIAN_POINT('Ctrl Pts',(-24.2499912798646,19.7521565392983,33.9947971375223)) ;
#10466=CARTESIAN_POINT('Ctrl Pts',(-24.2495525067901,19.7792823248453,33.9954915308927)) ;
#10467=CARTESIAN_POINT('Ctrl Pts',(-24.244045930543,19.8049989553455,33.9961569948495)) ;
#10468=CARTESIAN_POINT('Ctrl Pts',(-24.2234830661828,19.8528694600569,33.9974077124504)) ;
#10469=CARTESIAN_POINT('Ctrl Pts',(-24.2086245409041,19.8745668657937,33.997980931313)) ;
#10470=CARTESIAN_POINT('Ctrl Pts',(-24.1714290071766,19.9110377740365,33.9989510216977)) ;
#10471=CARTESIAN_POINT('Ctrl Pts',(-24.1494502192513,19.9254650423844,33.9993384812983)) ;
#10472=CARTESIAN_POINT('Ctrl Pts',(-24.1014008539367,19.944999534253,33.9998644932132)) ;
#10473=CARTESIAN_POINT('Ctrl Pts',(-24.0758210331691,19.95,34.)) ;
#10474=CARTESIAN_POINT('Ctrl Pts',(-24.05,19.95,34.0000000000001)) ;
#10475=CARTESIAN_POINT('Origin',(-24.05,19.75,10.512952685943)) ;
#10476=CARTESIAN_POINT('',(-24.25,19.75,10.512952685943)) ;
#10477=CARTESIAN_POINT('Origin',(-24.05,27.3698141664511,-1.38697145397653)) ;
#10478=CARTESIAN_POINT('',(-24.05,23.15,2.55)) ;
#10479=CARTESIAN_POINT('',(-24.25,23.2911535780143,2.69168913446027)) ;
#10480=CARTESIAN_POINT('Ctrl Pts',(-24.05,23.15,2.55)) ;
#10481=CARTESIAN_POINT('Ctrl Pts',(-24.0632701694843,23.1499886889779,2.55001131102213)) ;
#10482=CARTESIAN_POINT('Ctrl Pts',(-24.0765399924101,23.1509143468025,2.55095959089099)) ;
#10483=CARTESIAN_POINT('Ctrl Pts',(-24.0895481340208,23.1527585208895,2.55282638702233)) ;
#10484=CARTESIAN_POINT('Ctrl Pts',(-24.1025532968563,23.1546022726734,2.55469275567017)) ;
#10485=CARTESIAN_POINT('Ctrl Pts',(-24.1152962197139,23.1573640218908,2.55747712175156)) ;
#10486=CARTESIAN_POINT('Ctrl Pts',(-24.1275260588054,23.1609891810431,2.56112489776775)) ;
#10487=CARTESIAN_POINT('Ctrl Pts',(-24.1397534773072,23.164613622686,2.56477195179821)) ;
#10488=CARTESIAN_POINT('Ctrl Pts',(-24.1514673780365,23.1691009417701,2.56928188326987)) ;
#10489=CARTESIAN_POINT('Ctrl Pts',(-24.1624372641837,23.1743626179299,2.57456617181717)) ;
#10490=CARTESIAN_POINT('Ctrl Pts',(-24.1734053194262,23.1796234159013,2.57984957840199)) ;
#10491=CARTESIAN_POINT('Ctrl Pts',(-24.1836290375724,23.1856580368581,2.58590680797231)) ;
#10492=CARTESIAN_POINT('Ctrl Pts',(-24.1929073111898,23.1923475533722,2.59261893309988)) ;
#10493=CARTESIAN_POINT('Ctrl Pts',(-24.2021908572985,23.1990408712851,2.59933487247379)) ;
#10494=CARTESIAN_POINT('Ctrl Pts',(-24.2105273961138,23.2063894818443,2.60670610449407)) ;
#10495=CARTESIAN_POINT('Ctrl Pts',(-24.2177527569689,23.2142484468191,2.61458769092999)) ;
#10496=CARTESIAN_POINT('Ctrl Pts',(-24.2249750808544,23.2221041085074,2.62246596457109)) ;
#10497=CARTESIAN_POINT('Ctrl Pts',(-24.2310867869367,23.2304692838499,2.63085375186639)) ;
#10498=CARTESIAN_POINT('Ctrl Pts',(-24.2359676185276,23.2391791534182,2.63958623338751)) ;
#10499=CARTESIAN_POINT('Ctrl Pts',(-24.2408502551657,23.2478922441029,2.64832194438742)) ;
#10500=CARTESIAN_POINT('Ctrl Pts',(-24.2445008489509,23.2569498295499,2.65740215014967)) ;
#10501=CARTESIAN_POINT('Ctrl Pts',(-24.2468475163264,23.2661733348448,2.66664827575977)) ;
#10502=CARTESIAN_POINT('Ctrl Pts',(-24.2489436334282,23.2744120598512,2.67490720594314)) ;
#10503=CARTESIAN_POINT('Ctrl Pts',(-24.25,23.2827827492619,2.68329810053082)) ;
#10504=CARTESIAN_POINT('Ctrl Pts',(-24.25,23.2911535780144,2.6916891344603)) ;
#10505=CARTESIAN_POINT('',(-24.25,27.3698141664511,-1.38697145397653)) ;
#10506=CARTESIAN_POINT('',(-24.05,27.2283928102138,-1.52839281021384)) ;
#10507=CARTESIAN_POINT('Origin',(-24.05,17.2261159840305,33.8238840159695)) ;
#10508=CARTESIAN_POINT('',(-24.25,17.1987235045028,33.2996639834704)) ;
#10509=CARTESIAN_POINT('Origin',(-24.25,17.2261159840305,33.8238840159695)) ;
#10510=CARTESIAN_POINT('Ctrl Pts',(-24.25,17.1987235045028,33.2996639834704)) ;
#10511=CARTESIAN_POINT('Ctrl Pts',(-24.25,17.1987230610883,33.301013065151)) ;
#10512=CARTESIAN_POINT('Ctrl Pts',(-24.2499863874771,17.1987227661361,33.3023621127686)) ;
#10513=CARTESIAN_POINT('Ctrl Pts',(-24.2494407904293,17.1987198608847,33.3293950031184)) ;
#10514=CARTESIAN_POINT('Ctrl Pts',(-24.2439924301409,17.1987735623143,33.3547437391131)) ;
#10515=CARTESIAN_POINT('Ctrl Pts',(-24.2236773306868,17.1989855389576,33.4023588449877)) ;
#10516=CARTESIAN_POINT('Ctrl Pts',(-24.2088610786989,17.1991433664022,33.4241220030844)) ;
#10517=CARTESIAN_POINT('Ctrl Pts',(-24.1717621164808,17.199483617429,33.4607013743553)) ;
#10518=CARTESIAN_POINT('Ctrl Pts',(-24.1498475303235,17.1996607603534,33.475185047544)) ;
#10519=CARTESIAN_POINT('Ctrl Pts',(-24.1017273992471,17.199921556701,33.4949236590357)) ;
#10520=CARTESIAN_POINT('Ctrl Pts',(-24.0759897994102,17.2,33.5)) ;
#10521=CARTESIAN_POINT('Ctrl Pts',(-24.05,17.2,33.5)) ;
#10522=CARTESIAN_POINT('Origin',(-24.05,20.3521649222088,3.15764237037056)) ;
#10523=CARTESIAN_POINT('',(-24.25,18.2941489582325,11.498022857368)) ;
#10524=CARTESIAN_POINT('',(-24.25,20.3521649222088,3.15764237037056)) ;
#10525=CARTESIAN_POINT('',(-24.05,18.1,11.45)) ;
#10526=CARTESIAN_POINT('Ctrl Pts',(-24.25,18.2941488864464,11.4980231468816)) ;
#10527=CARTESIAN_POINT('Ctrl Pts',(-24.25,18.2931711440881,11.4977812986393)) ;
#10528=CARTESIAN_POINT('Ctrl Pts',(-24.2499923914673,18.292193415111,11.4975394541043)) ;
#10529=CARTESIAN_POINT('Ctrl Pts',(-24.2495857492044,18.2660672742236,11.491077053847)) ;
#10530=CARTESIAN_POINT('Ctrl Pts',(-24.2441638802667,18.2412305566091,11.4849336180087)) ;
#10531=CARTESIAN_POINT('Ctrl Pts',(-24.2238111338179,18.1948292452196,11.4734561374442)) ;
#10532=CARTESIAN_POINT('Ctrl Pts',(-24.2090259631664,18.173725801069,11.4682361612198)) ;
#10533=CARTESIAN_POINT('Ctrl Pts',(-24.1719547805075,18.1382083382914,11.4594508639049)) ;
#10534=CARTESIAN_POINT('Ctrl Pts',(-24.1500231903924,18.1241338849213,11.4559695344032)) ;
#10535=CARTESIAN_POINT('Ctrl Pts',(-24.1018369369122,18.104937954276,11.4512214053055)) ;
#10536=CARTESIAN_POINT('Ctrl Pts',(-24.0760429610237,18.0999999999997,11.4500000000011)) ;
#10537=CARTESIAN_POINT('Ctrl Pts',(-24.05,18.0999999999997,11.4500000000014)) ;
#10538=CARTESIAN_POINT('',(-24.05,20.1579889903124,3.10972882873379)) ;
#10539=CARTESIAN_POINT('Origin',(-24.05,36.5141483124065,16.0157526941183)) ;
#10540=CARTESIAN_POINT('Origin',(-24.05,36.5141483124065,16.0157526941183)) ;
#10541=CARTESIAN_POINT('Origin',(-24.25,36.5141483124065,16.0157526941183)) ;
#10542=CARTESIAN_POINT('Origin',(-24.05,17.5172318824408,27.2801860892852)) ;
#10543=CARTESIAN_POINT('',(-24.25,11.9761936845669,29.6534659706104)) ;
#10544=CARTESIAN_POINT('Origin',(-24.25,17.5172318824408,27.2801860892852)) ;
#10545=CARTESIAN_POINT('Ctrl Pts',(-24.25,11.976193684567,29.6534659706103)) ;
#10546=CARTESIAN_POINT('Ctrl Pts',(-24.25,11.9755977818072,29.6537918503201)) ;
#10547=CARTESIAN_POINT('Ctrl Pts',(-24.249996571899,11.9750018853708,29.6541177328252)) ;
#10548=CARTESIAN_POINT('Ctrl Pts',(-24.2497216151694,11.9511052235039,29.6671865363954)) ;
#10549=CARTESIAN_POINT('Ctrl Pts',(-24.2442143166798,11.9280772247116,29.67979017374)) ;
#10550=CARTESIAN_POINT('Ctrl Pts',(-24.2235106312593,11.8855929764579,29.7030577904185)) ;
#10551=CARTESIAN_POINT('Ctrl Pts',(-24.2086691696459,11.866481196583,29.7135326615679)) ;
#10552=CARTESIAN_POINT('Ctrl Pts',(-24.1715506168807,11.8344052888093,29.7311205240322)) ;
#10553=CARTESIAN_POINT('Ctrl Pts',(-24.1496614544952,11.8217190498113,29.7380808841414)) ;
#10554=CARTESIAN_POINT('Ctrl Pts',(-24.1016151251543,11.8044416410205,29.7475617250063)) ;
#10555=CARTESIAN_POINT('Ctrl Pts',(-24.0759347764714,11.8,29.75)) ;
#10556=CARTESIAN_POINT('Ctrl Pts',(-24.05,11.8,29.75)) ;
#10557=CARTESIAN_POINT('Origin',(-24.05,3.95376271603246,17.8309361222439)) ;
#10558=CARTESIAN_POINT('',(-24.25,11.0061123301193,28.2238723956349)) ;
#10559=CARTESIAN_POINT('',(-24.25,3.95376271603246,17.8309361222439)) ;
#10560=CARTESIAN_POINT('Ctrl Pts',(-24.25,11.0061123301191,28.2238723956351)) ;
#10561=CARTESIAN_POINT('Ctrl Pts',(-24.25,11.0055804043094,28.2243014934111)) ;
#10562=CARTESIAN_POINT('Ctrl Pts',(-24.2499965208248,11.0050484851104,28.2247305924736)) ;
#10563=CARTESIAN_POINT('Ctrl Pts',(-24.24971885402,10.9838233720669,28.24185314932)) ;
#10564=CARTESIAN_POINT('Ctrl Pts',(-24.2441849834891,10.9633766729638,28.2583581483305)) ;
#10565=CARTESIAN_POINT('Ctrl Pts',(-24.2234123635662,10.92570478066,28.2887842809354)) ;
#10566=CARTESIAN_POINT('Ctrl Pts',(-24.2085470530348,10.908781248086,28.3024612708704)) ;
#10567=CARTESIAN_POINT('Ctrl Pts',(-24.1713793201344,10.8803789404798,28.3254235047367)) ;
#10568=CARTESIAN_POINT('Ctrl Pts',(-24.1494579257414,10.8691509765059,28.3345056873335)) ;
#10569=CARTESIAN_POINT('Ctrl Pts',(-24.101449145542,10.8539092421029,28.3468363151276)) ;
#10570=CARTESIAN_POINT('Ctrl Pts',(-24.0758491730085,10.85,28.35)) ;
#10571=CARTESIAN_POINT('Ctrl Pts',(-24.05,10.85,28.35)) ;
#10572=CARTESIAN_POINT('Origin',(-24.05,6.94557266623349,32.0941410006498)) ;
#10573=CARTESIAN_POINT('',(-24.25,8.97014939515615,26.8626927780581)) ;
#10574=CARTESIAN_POINT('Origin',(-24.25,6.94557266623349,32.0941410006498)) ;
#10575=CARTESIAN_POINT('Ctrl Pts',(-24.25,8.97014939515615,26.8626927780581)) ;
#10576=CARTESIAN_POINT('Ctrl Pts',(-24.25,8.96980308364487,26.8636177522324)) ;
#10577=CARTESIAN_POINT('Ctrl Pts',(-24.2499926845694,8.96945677554181,26.8645427132223)) ;
#10578=CARTESIAN_POINT('Ctrl Pts',(-24.2495939082893,8.96001834118659,26.8897518974775)) ;
#10579=CARTESIAN_POINT('Ctrl Pts',(-24.2441704958547,8.95103756375155,26.9137357983753)) ;
#10580=CARTESIAN_POINT('Ctrl Pts',(-24.2238069800194,8.93426601854433,26.9585208446484)) ;
#10581=CARTESIAN_POINT('Ctrl Pts',(-24.2090209946366,8.92664079883623,26.9788799538848)) ;
#10582=CARTESIAN_POINT('Ctrl Pts',(-24.1719491121253,8.91380708303496,27.0131430696368)) ;
#10583=CARTESIAN_POINT('Ctrl Pts',(-24.1500181006065,8.90872114416501,27.0267199513304)) ;
#10584=CARTESIAN_POINT('Ctrl Pts',(-24.1018338032566,8.90178447987708,27.0452368074564)) ;
#10585=CARTESIAN_POINT('Ctrl Pts',(-24.0760414340743,8.90000000000021,27.0500000000001)) ;
#10586=CARTESIAN_POINT('Ctrl Pts',(-24.05,8.9000000000002,27.0500000000001)) ;
#10587=CARTESIAN_POINT('Origin',(-24.05,9.21323262385133,26.950665756062)) ;
#10588=CARTESIAN_POINT('',(-24.25,3.70650846391516,24.9577560600852)) ;
#10589=CARTESIAN_POINT('',(-24.25,9.21323262385133,26.950665756062)) ;
#10590=CARTESIAN_POINT('Ctrl Pts',(-24.25,3.70650846391515,24.9577560600852)) ;
#10591=CARTESIAN_POINT('Ctrl Pts',(-24.25,3.70613263983912,24.9591249412748)) ;
#10592=CARTESIAN_POINT('Ctrl Pts',(-24.2499849817197,3.70575595542866,24.9604935443132)) ;
#10593=CARTESIAN_POINT('Ctrl Pts',(-24.249412424472,3.69856163593084,24.9865707375015)) ;
#10594=CARTESIAN_POINT('Ctrl Pts',(-24.243975112071,3.69157540066717,25.0108789195625)) ;
#10595=CARTESIAN_POINT('Ctrl Pts',(-24.2237007313829,3.67823129499148,25.0565205811117)) ;
#10596=CARTESIAN_POINT('Ctrl Pts',(-24.2089065576862,3.67201058953836,25.0773585750523)) ;
#10597=CARTESIAN_POINT('Ctrl Pts',(-24.1718321061545,3.66147275373824,25.1123866592332)) ;
#10598=CARTESIAN_POINT('Ctrl Pts',(-24.1499165688336,3.65725415494464,25.1262472800193)) ;
#10599=CARTESIAN_POINT('Ctrl Pts',(-24.1017741331367,3.65149079158464,25.1451425855635)) ;
#10600=CARTESIAN_POINT('Ctrl Pts',(-24.0760121197655,3.64999999999993,25.15)) ;
#10601=CARTESIAN_POINT('Ctrl Pts',(-24.05,3.64999999999994,25.15)) ;
#10602=CARTESIAN_POINT('Ctrl Pts',(-24.25,3.70650846391516,24.9577560600852)) ;
#10603=CARTESIAN_POINT('Ctrl Pts',(-24.25,3.58356237630651,24.9342829362711)) ;
#10604=CARTESIAN_POINT('Ctrl Pts',(-24.25,3.6,24.8102001714438)) ;
#10605=CARTESIAN_POINT('Ctrl Pts',(-24.25,3.66900151529777,25.1542076541367)) ;
#10606=CARTESIAN_POINT('Ctrl Pts',(-24.25,3.36048403150656,25.0953048518053)) ;
#10607=CARTESIAN_POINT('Ctrl Pts',(-24.25,3.40173214602618,24.7839350218989)) ;
#10608=CARTESIAN_POINT('Ctrl Pts',(-24.05,3.66900151529777,25.1542076541367)) ;
#10609=CARTESIAN_POINT('Ctrl Pts',(-24.05,3.36048403150656,25.0953048518053)) ;
#10610=CARTESIAN_POINT('Ctrl Pts',(-24.05,3.40173214602618,24.7839350218989)) ;
#10611=CARTESIAN_POINT('',(-24.25,3.6,24.8102001714438)) ;
#10612=CARTESIAN_POINT('Origin',(-24.25,3.73135783556136,24.8276015460276)) ;
#10613=CARTESIAN_POINT('Ctrl Pts',(-24.25,3.6,24.8102001714438)) ;
#10614=CARTESIAN_POINT('Ctrl Pts',(-24.25,3.59858329627815,24.8101067420225)) ;
#10615=CARTESIAN_POINT('Ctrl Pts',(-24.2499849471218,3.59716658347762,24.8100140642959)) ;
#10616=CARTESIAN_POINT('Ctrl Pts',(-24.2494121494215,3.57021683344487,24.8082647222741)) ;
#10617=CARTESIAN_POINT('Ctrl Pts',(-24.2439829942548,3.54500851791206,24.8068523074975)) ;
#10618=CARTESIAN_POINT('Ctrl Pts',(-24.2237349857366,3.49756309113979,24.8043748002524)) ;
#10619=CARTESIAN_POINT('Ctrl Pts',(-24.2089435980113,3.4758431175171,24.8033431470145)) ;
#10620=CARTESIAN_POINT('Ctrl Pts',(-24.1718701468162,3.43929965309513,24.801671969686)) ;
#10621=CARTESIAN_POINT('Ctrl Pts',(-24.1499496297251,3.42482149959621,24.8010487344218)) ;
#10622=CARTESIAN_POINT('Ctrl Pts',(-24.1017936039468,3.40507852591201,24.8002087457528)) ;
#10623=CARTESIAN_POINT('Ctrl Pts',(-24.0760216817082,3.4,24.8)) ;
#10624=CARTESIAN_POINT('Ctrl Pts',(-24.05,3.4,24.8)) ;
#10625=CARTESIAN_POINT('Origin',(-24.05,3.6,5.91295268594296)) ;
#10626=CARTESIAN_POINT('',(-24.25,3.6,5.91295268594296)) ;
#10627=CARTESIAN_POINT('Origin',(-24.25,3.9,19.5)) ;
#10628=CARTESIAN_POINT('',(-24.25,10.8,22.)) ;
#10629=CARTESIAN_POINT('Origin',(-24.25,12.2182755082439,18.0689260404997)) ;
#10630=CARTESIAN_POINT('',(-24.25,12.85,22.2)) ;
#10631=CARTESIAN_POINT('Origin',(-24.25,12.85,22.2)) ;
#10632=CARTESIAN_POINT('',(-24.25,15.5,20.65)) ;
#10633=CARTESIAN_POINT('Origin',(-24.25,12.5256959686759,18.3486581187154)) ;
#10634=CARTESIAN_POINT('',(-24.25,16.2,19.15)) ;
#10635=CARTESIAN_POINT('Origin',(-24.25,16.2,19.15)) ;
#10636=CARTESIAN_POINT('',(-24.25,18.1,11.45)) ;
#10637=CARTESIAN_POINT('Origin',(-24.25,36.5141483124065,16.0157526941183)) ;
#10638=CARTESIAN_POINT('',(-24.25,23.15,2.55)) ;
#10639=CARTESIAN_POINT('Origin',(-24.25,23.15,2.55)) ;
#10640=CARTESIAN_POINT('',(-24.25,35.4,-9.7)) ;
#10641=CARTESIAN_POINT('Origin',(-24.25,29.7633733578399,-15.291248496029)) ;
#10642=CARTESIAN_POINT('',(-24.25,37.7,-15.5)) ;
#10643=CARTESIAN_POINT('Origin',(-24.25,37.7,-15.5)) ;
#10644=CARTESIAN_POINT('',(-24.25,36.65,-56.2)) ;
#10645=CARTESIAN_POINT('Origin',(-24.25,37.7318176617063,-60.502128268216)) ;
#10646=CARTESIAN_POINT('',(-24.25,42.15,-60.9)) ;
#10647=CARTESIAN_POINT('Origin',(-24.25,42.15,-60.9)) ;
#10648=CARTESIAN_POINT('',(-24.25,42.3,-58.75)) ;
#10649=CARTESIAN_POINT('Origin',(-24.25,42.3,-58.75)) ;
#10650=CARTESIAN_POINT('',(-24.25,44.45,-17.3)) ;
#10651=CARTESIAN_POINT('Origin',(-24.25,23.7122919887408,-16.1822567109578)) ;
#10652=CARTESIAN_POINT('',(-24.25,38.35,-1.45)) ;
#10653=CARTESIAN_POINT('Origin',(-24.25,38.35,-1.45)) ;
#10654=CARTESIAN_POINT('Origin',(-24.25,23.9394766127413,-12.9740946281141)) ;
#10655=CARTESIAN_POINT('',(-24.25,19.6,36.797821691004)) ;
#10656=CARTESIAN_POINT('',(-24.25,17.9,36.797821691004)) ;
#10657=CARTESIAN_POINT('Origin',(-24.25,18.75,36.8151771653543)) ;
#10658=CARTESIAN_POINT('',(-24.25,19.6,37.802178308996)) ;
#10659=CARTESIAN_POINT('',(-24.25,19.6,12.412952685943)) ;
#10660=CARTESIAN_POINT('',(-24.25,17.9,37.802178308996)) ;
#10661=CARTESIAN_POINT('Origin',(-24.25,18.75,37.7848228346457)) ;
#10662=CARTESIAN_POINT('',(-24.25,17.9,11.912952685943)) ;
#10663=CARTESIAN_POINT('',(-24.25,17.565,31.11)) ;
#10664=CARTESIAN_POINT('Origin',(-24.25,17.565,27.14)) ;
#10665=CARTESIAN_POINT('Origin',(-16.5,19.6,12.412952685943)) ;
#10666=CARTESIAN_POINT('',(-16.5,19.4,37.8)) ;
#10667=CARTESIAN_POINT('Ctrl Pts',(-16.3,19.6,37.802178308996)) ;
#10668=CARTESIAN_POINT('Ctrl Pts',(-16.3,19.5980557067222,37.8021584615749)) ;
#10669=CARTESIAN_POINT('Ctrl Pts',(-16.3000283520726,19.5961115171112,37.8021385811547)) ;
#10670=CARTESIAN_POINT('Ctrl Pts',(-16.3008130702058,19.5692119515023,37.8018630425845)) ;
#10671=CARTESIAN_POINT('Ctrl Pts',(-16.3062077376902,19.544611369092,37.8016051814373)) ;
#10672=CARTESIAN_POINT('Ctrl Pts',(-16.3261931704212,19.4976798310454,37.8011023681781)) ;
#10673=CARTESIAN_POINT('Ctrl Pts',(-16.3409792801415,19.4759408829566,37.8008632966273)) ;
#10674=CARTESIAN_POINT('Ctrl Pts',(-16.378051291451,19.4393554460034,37.8004539917046)) ;
#10675=CARTESIAN_POINT('Ctrl Pts',(-16.3999823105663,19.4248582008503,37.8002878723196)) ;
#10676=CARTESIAN_POINT('Ctrl Pts',(-16.4481664789317,19.4050861143264,37.8000596824773)) ;
#10677=CARTESIAN_POINT('Ctrl Pts',(-16.4739586994907,19.4,37.8)) ;
#10678=CARTESIAN_POINT('Ctrl Pts',(-16.5,19.4,37.8)) ;
#10679=CARTESIAN_POINT('',(-16.5,19.4,36.8)) ;
#10680=CARTESIAN_POINT('',(-16.5,19.4,12.412952685943)) ;
#10681=CARTESIAN_POINT('Ctrl Pts',(-16.3,19.6,36.797821691004)) ;
#10682=CARTESIAN_POINT('Ctrl Pts',(-16.3,19.5980557067222,36.797841538425)) ;
#10683=CARTESIAN_POINT('Ctrl Pts',(-16.3000283520726,19.5961115171112,36.7978614188453)) ;
#10684=CARTESIAN_POINT('Ctrl Pts',(-16.3008130702058,19.5692119515023,36.7981369574155)) ;
#10685=CARTESIAN_POINT('Ctrl Pts',(-16.3062077376902,19.544611369092,36.7983948185627)) ;
#10686=CARTESIAN_POINT('Ctrl Pts',(-16.3261931704212,19.4976798310454,36.7988976318219)) ;
#10687=CARTESIAN_POINT('Ctrl Pts',(-16.3409792801416,19.4759408829566,36.7991367033726)) ;
#10688=CARTESIAN_POINT('Ctrl Pts',(-16.3780512914511,19.4393554460034,36.7995460082953)) ;
#10689=CARTESIAN_POINT('Ctrl Pts',(-16.3999823105663,19.4248582008503,36.7997121276805)) ;
#10690=CARTESIAN_POINT('Ctrl Pts',(-16.4481664789317,19.4050861143264,36.7999403175228)) ;
#10691=CARTESIAN_POINT('Ctrl Pts',(-16.4739586994907,19.4,36.8)) ;
#10692=CARTESIAN_POINT('Ctrl Pts',(-16.5,19.4,36.8)) ;
#10693=CARTESIAN_POINT('Origin',(-16.5,18.75,37.7848228346457)) ;
#10694=CARTESIAN_POINT('',(-16.5,18.1,37.8)) ;
#10695=CARTESIAN_POINT('Ctrl Pts',(-16.3,17.9,37.8021783089959)) ;
#10696=CARTESIAN_POINT('Ctrl Pts',(-16.3,17.9019442932778,37.8021584615748)) ;
#10697=CARTESIAN_POINT('Ctrl Pts',(-16.3000283520726,17.9038884828888,37.8021385811547)) ;
#10698=CARTESIAN_POINT('Ctrl Pts',(-16.3008130702058,17.9307880484977,37.8018630425845)) ;
#10699=CARTESIAN_POINT('Ctrl Pts',(-16.3062077376903,17.9553886309081,37.8016051814374)) ;
#10700=CARTESIAN_POINT('Ctrl Pts',(-16.3261931704213,18.0023201689547,37.8011023681781)) ;
#10701=CARTESIAN_POINT('Ctrl Pts',(-16.3409792801416,18.0240591170434,37.8008632966274)) ;
#10702=CARTESIAN_POINT('Ctrl Pts',(-16.3780512914511,18.0606445539966,37.8004539917047)) ;
#10703=CARTESIAN_POINT('Ctrl Pts',(-16.3999823105663,18.0751417991497,37.8002878723196)) ;
#10704=CARTESIAN_POINT('Ctrl Pts',(-16.4481664789317,18.0949138856736,37.8000596824773)) ;
#10705=CARTESIAN_POINT('Ctrl Pts',(-16.4739586994907,18.1,37.8)) ;
#10706=CARTESIAN_POINT('Ctrl Pts',(-16.5,18.1,37.8)) ;
#10707=CARTESIAN_POINT('Origin',(-16.5,18.75,37.7848228346457)) ;
#10708=CARTESIAN_POINT('Origin',(-16.5,17.9,11.912952685943)) ;
#10709=CARTESIAN_POINT('',(-16.5,18.1,36.8)) ;
#10710=CARTESIAN_POINT('Ctrl Pts',(-16.3,17.9,36.797821691004)) ;
#10711=CARTESIAN_POINT('Ctrl Pts',(-16.3,17.9019442932778,36.7978415384251)) ;
#10712=CARTESIAN_POINT('Ctrl Pts',(-16.3000283520726,17.9038884828888,36.7978614188453)) ;
#10713=CARTESIAN_POINT('Ctrl Pts',(-16.3008130702058,17.9307880484976,36.7981369574155)) ;
#10714=CARTESIAN_POINT('Ctrl Pts',(-16.3062077376902,17.955388630908,36.7983948185627)) ;
#10715=CARTESIAN_POINT('Ctrl Pts',(-16.3261931704212,18.0023201689546,36.7988976318219)) ;
#10716=CARTESIAN_POINT('Ctrl Pts',(-16.3409792801416,18.0240591170434,36.7991367033726)) ;
#10717=CARTESIAN_POINT('Ctrl Pts',(-16.3780512914511,18.0606445539966,36.7995460082953)) ;
#10718=CARTESIAN_POINT('Ctrl Pts',(-16.3999823105663,18.0751417991497,36.7997121276805)) ;
#10719=CARTESIAN_POINT('Ctrl Pts',(-16.4481664789317,18.0949138856736,36.7999403175228)) ;
#10720=CARTESIAN_POINT('Ctrl Pts',(-16.4739586994907,18.1,36.8)) ;
#10721=CARTESIAN_POINT('Ctrl Pts',(-16.5,18.1,36.8)) ;
#10722=CARTESIAN_POINT('',(-16.5,18.1,11.912952685943)) ;
#10723=CARTESIAN_POINT('Origin',(-16.5,18.75,36.8151771653543)) ;
#10724=CARTESIAN_POINT('Origin',(-16.5,18.75,36.8151771653543)) ;
#10725=CARTESIAN_POINT('Origin',(-24.25,18.75,36.8151771653543)) ;
#10726=CARTESIAN_POINT('',(-24.05,19.4,36.8)) ;
#10727=CARTESIAN_POINT('',(-24.25,19.4,36.8)) ;
#10728=CARTESIAN_POINT('',(-24.05,18.1,36.8)) ;
#10729=CARTESIAN_POINT('Origin',(-24.05,18.75,36.8151771653543)) ;
#10730=CARTESIAN_POINT('',(-24.25,18.1,36.8)) ;
#10731=CARTESIAN_POINT('Origin',(-24.25,19.4,37.8)) ;
#10732=CARTESIAN_POINT('',(-24.05,19.4,37.8)) ;
#10733=CARTESIAN_POINT('',(-24.25,19.4,37.8)) ;
#10734=CARTESIAN_POINT('',(-24.05,19.4,12.412952685943)) ;
#10735=CARTESIAN_POINT('Origin',(-24.05,18.75,37.7848228346457)) ;
#10736=CARTESIAN_POINT('',(-24.05,18.1,37.8)) ;
#10737=CARTESIAN_POINT('Origin',(-24.05,18.75,37.7848228346457)) ;
#10738=CARTESIAN_POINT('Ctrl Pts',(-24.05,18.1,37.8)) ;
#10739=CARTESIAN_POINT('Ctrl Pts',(-24.0760413005093,18.1,37.8)) ;
#10740=CARTESIAN_POINT('Ctrl Pts',(-24.1018335210683,18.0949138856736,37.8000596824775)) ;
#10741=CARTESIAN_POINT('Ctrl Pts',(-24.1500176894337,18.0751417991497,37.8002878723198)) ;
#10742=CARTESIAN_POINT('Ctrl Pts',(-24.171948708549,18.0606445539966,37.8004539917047)) ;
#10743=CARTESIAN_POINT('Ctrl Pts',(-24.2090207198584,18.0240591170434,37.8008632966275)) ;
#10744=CARTESIAN_POINT('Ctrl Pts',(-24.2238068295788,18.0023201689546,37.801102368178)) ;
#10745=CARTESIAN_POINT('Ctrl Pts',(-24.2437922623098,17.9553886309081,37.8016051814372)) ;
#10746=CARTESIAN_POINT('Ctrl Pts',(-24.2491869297942,17.9307880484976,37.8018630425845)) ;
#10747=CARTESIAN_POINT('Ctrl Pts',(-24.2499716479274,17.9038884828888,37.8021385811547)) ;
#10748=CARTESIAN_POINT('Ctrl Pts',(-24.25,17.9019442932778,37.8021584615749)) ;
#10749=CARTESIAN_POINT('Ctrl Pts',(-24.25,17.9,37.802178308996)) ;
#10750=CARTESIAN_POINT('Ctrl Pts',(-24.25,19.6,37.802178308996)) ;
#10751=CARTESIAN_POINT('Ctrl Pts',(-24.25,19.5980557067222,37.8021584615749)) ;
#10752=CARTESIAN_POINT('Ctrl Pts',(-24.2499716479274,19.5961115171112,37.8021385811546)) ;
#10753=CARTESIAN_POINT('Ctrl Pts',(-24.2491869297942,19.5692119515024,37.8018630425845)) ;
#10754=CARTESIAN_POINT('Ctrl Pts',(-24.2437922623098,19.5446113690919,37.801605181438)) ;
#10755=CARTESIAN_POINT('Ctrl Pts',(-24.2238068295787,19.4976798310453,37.8011023681784)) ;
#10756=CARTESIAN_POINT('Ctrl Pts',(-24.2090207198584,19.4759408829566,37.8008632966275)) ;
#10757=CARTESIAN_POINT('Ctrl Pts',(-24.171948708549,19.4393554460034,37.8004539917047)) ;
#10758=CARTESIAN_POINT('Ctrl Pts',(-24.1500176894337,19.4248582008503,37.8002878723198)) ;
#10759=CARTESIAN_POINT('Ctrl Pts',(-24.1018335210683,19.4050861143264,37.8000596824775)) ;
#10760=CARTESIAN_POINT('Ctrl Pts',(-24.0760413005093,19.4,37.8)) ;
#10761=CARTESIAN_POINT('Ctrl Pts',(-24.05,19.4,37.8)) ;
#10762=CARTESIAN_POINT('Origin',(-24.05,18.75,36.8151771653543)) ;
#10763=CARTESIAN_POINT('Ctrl Pts',(-24.25,17.9,36.797821691004)) ;
#10764=CARTESIAN_POINT('Ctrl Pts',(-24.25,17.9019442932778,36.7978415384251)) ;
#10765=CARTESIAN_POINT('Ctrl Pts',(-24.2499716479274,17.9038884828888,36.7978614188453)) ;
#10766=CARTESIAN_POINT('Ctrl Pts',(-24.2491869297942,17.9307880484977,36.7981369574155)) ;
#10767=CARTESIAN_POINT('Ctrl Pts',(-24.2437922623098,17.9553886309081,36.7983948185627)) ;
#10768=CARTESIAN_POINT('Ctrl Pts',(-24.2238068295788,18.0023201689546,36.798897631822)) ;
#10769=CARTESIAN_POINT('Ctrl Pts',(-24.2090207198584,18.0240591170434,36.7991367033725)) ;
#10770=CARTESIAN_POINT('Ctrl Pts',(-24.171948708549,18.0606445539966,36.7995460082953)) ;
#10771=CARTESIAN_POINT('Ctrl Pts',(-24.1500176894337,18.0751417991497,36.7997121276803)) ;
#10772=CARTESIAN_POINT('Ctrl Pts',(-24.1018335210683,18.0949138856736,36.7999403175226)) ;
#10773=CARTESIAN_POINT('Ctrl Pts',(-24.0760413005093,18.1,36.8)) ;
#10774=CARTESIAN_POINT('Ctrl Pts',(-24.05,18.1,36.8)) ;
#10775=CARTESIAN_POINT('Ctrl Pts',(-24.25,19.6,36.797821691004)) ;
#10776=CARTESIAN_POINT('Ctrl Pts',(-24.25,19.5980557067222,36.7978415384251)) ;
#10777=CARTESIAN_POINT('Ctrl Pts',(-24.2499716479274,19.5961115171112,36.7978614188453)) ;
#10778=CARTESIAN_POINT('Ctrl Pts',(-24.2491869297942,19.5692119515023,36.7981369574155)) ;
#10779=CARTESIAN_POINT('Ctrl Pts',(-24.2437922623098,19.5446113690919,36.7983948185627)) ;
#10780=CARTESIAN_POINT('Ctrl Pts',(-24.2238068295788,19.4976798310454,36.798897631822)) ;
#10781=CARTESIAN_POINT('Ctrl Pts',(-24.2090207198584,19.4759408829566,36.7991367033725)) ;
#10782=CARTESIAN_POINT('Ctrl Pts',(-24.171948708549,19.4393554460034,36.7995460082953)) ;
#10783=CARTESIAN_POINT('Ctrl Pts',(-24.1500176894337,19.4248582008503,36.7997121276803)) ;
#10784=CARTESIAN_POINT('Ctrl Pts',(-24.1018335210683,19.4050861143264,36.7999403175226)) ;
#10785=CARTESIAN_POINT('Ctrl Pts',(-24.0760413005093,19.4,36.8)) ;
#10786=CARTESIAN_POINT('Ctrl Pts',(-24.05,19.4,36.8)) ;
#10787=CARTESIAN_POINT('Origin',(-24.05,17.9,11.912952685943)) ;
#10788=CARTESIAN_POINT('',(-24.05,18.1,11.912952685943)) ;
#10789=CARTESIAN_POINT('Origin',(-24.05,19.6,12.412952685943)) ;
#10790=CARTESIAN_POINT('Origin',(-24.25,17.565,27.14)) ;
#10791=CARTESIAN_POINT('',(-24.25,17.565,31.11)) ;
#10792=CARTESIAN_POINT('Origin',(-24.25,18.1,36.8)) ;
#10793=CARTESIAN_POINT('',(-24.25,18.1,37.8)) ;
#10794=CARTESIAN_POINT('Origin',(-24.25,18.75,37.7848228346457)) ;
#11366=UNCERTAINTY_MEASURE_WITH_UNIT(LENGTH_MEASURE(0.01),#11397,
'DISTANCE_ACCURACY_VALUE',
'Maximum model space distance between geometric entities at asserted c
onnectivities') ;
#11379=UNCERTAINTY_MEASURE_WITH_UNIT(LENGTH_MEASURE(0.01),#11397,
'DISTANCE_ACCURACY_VALUE',
'Maximum model space distance between geometric entities at asserted c
onnectivities') ;
#11383=(
GEOMETRIC_REPRESENTATION_CONTEXT(3)
GLOBAL_UNCERTAINTY_ASSIGNED_CONTEXT((#11366))
GLOBAL_UNIT_ASSIGNED_CONTEXT((#11397,#11399,#11400))
REPRESENTATION_CONTEXT('','3D')
) ;
#11396=(
GEOMETRIC_REPRESENTATION_CONTEXT(3)
GLOBAL_UNCERTAINTY_ASSIGNED_CONTEXT((#11379))
GLOBAL_UNIT_ASSIGNED_CONTEXT((#11397,#11399,#11400))
REPRESENTATION_CONTEXT('','3D')
) ;
#11397=(
LENGTH_UNIT()
NAMED_UNIT(*)
SI_UNIT(.MILLI.,.METRE.)
) ;
#11399=(
NAMED_UNIT(*)
PLANE_ANGLE_UNIT()
SI_UNIT($,.RADIAN.)
) ;
#11400=(
NAMED_UNIT(*)
SI_UNIT($,.STERADIAN.)
SOLID_ANGLE_UNIT()
) ;
#11404=SHAPE_DEFINITION_REPRESENTATION(#11420,#11457) ;
#11420=PRODUCT_DEFINITION_SHAPE('',$,#11474) ;
#11457=SHAPE_REPRESENTATION('',(#6038),#11383) ;
#11470=PRODUCT_DEFINITION_CONTEXT('part definition',#11520,'design') ;
#11474=PRODUCT_DEFINITION('Lever Handle','Lever Handle',#11490,
#11470) ;
#11490=PRODUCT_DEFINITION_FORMATION('',$,#11525) ;
#11520=APPLICATION_CONTEXT(
'Core Data for Automotive Mechanical Design Process') ;
#11521=PRODUCT_CONTEXT('part definition',#11520,'mechanical') ;
#11525=PRODUCT('Lever Handle','Lever Handle',$,(#11521)) ;
#11541=PRESENTATION_STYLE_ASSIGNMENT((#11557)) ;
#11557=SURFACE_STYLE_USAGE(.BOTH.,#11573) ;
#11573=SURFACE_SIDE_STYLE('',(#11589)) ;
#11589=SURFACE_STYLE_FILL_AREA(#11605) ;
#11605=FILL_AREA_STYLE('MAS-252 Grey Paint - Lever Handle',(#11621)) ;
#11621=FILL_AREA_STYLE_COLOUR('MAS-252 Grey Paint - Lever Handle',#11637) ;
#11637=COLOUR_RGB('MAS-252 Grey Paint - Lever Handle', 0.31764706, 0.68627451, 0.89019608) ;
ENDSEC;
END-ISO-10303-21;
